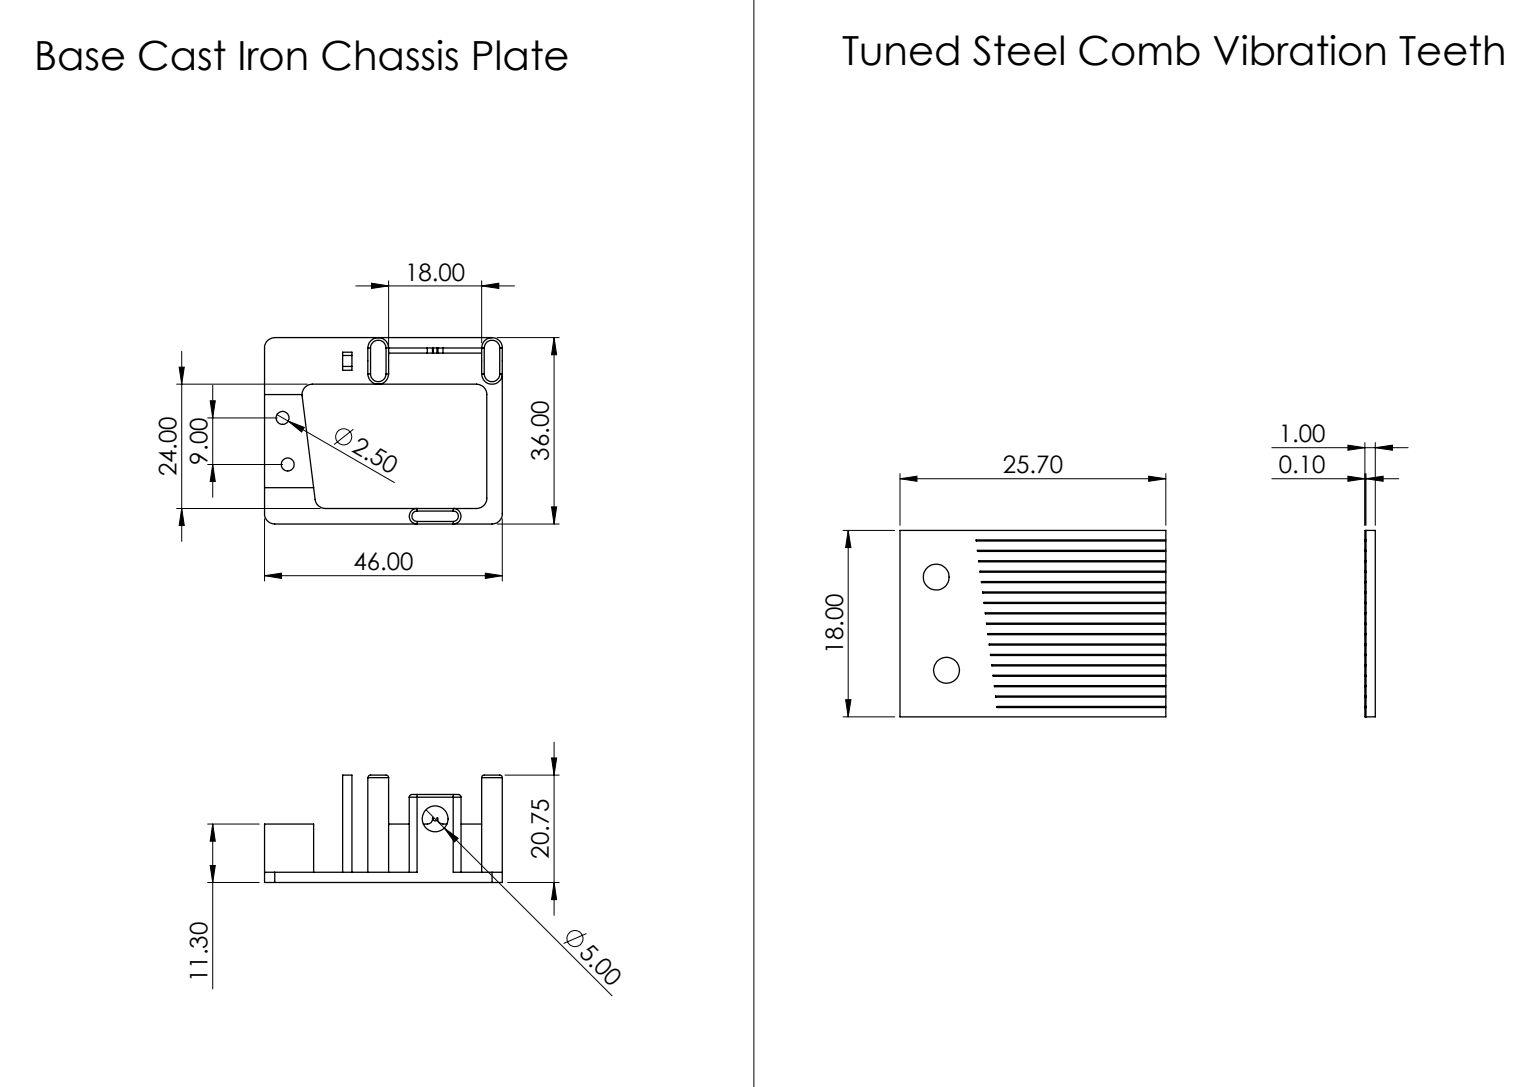
ISO-10303-21;
HEADER;
FILE_DESCRIPTION (('STEP AP214'),
    '1' );
FILE_NAME ('Tuned Steel Comb Vibration Teeth.step',
    '2026-10-09T09:51:18',
    ( '' ),
    ( '' ),
    'SwSTEP 2.0',
    'SolidWorks 2026',
    '' );
FILE_SCHEMA (( 'AUTOMOTIVE_DESIGN' ));
ENDSEC;

DATA;
#16=PLANE ( 'NONE',  #21145 ) ;
#64=LINE ( 'NONE', #7461, #9828 ) ;
#76=MANIFOLD_SOLID_BREP ( 'Stock-MAS-175-1', #12603 ) ;
#123=AXIS2_PLACEMENT_3D ( 'NONE', #20425, #35422, #737 ) ;
#135=ORIENTED_EDGE ( 'NONE', *, *, #41849, .T. ) ;
#167=CARTESIAN_POINT ( 'NONE',  ( -24.72409385541305582, -14.80920654474425291, 71.08235294117645253 ) ) ;
#180=DIRECTION ( 'NONE',  ( -2.866981220435666553E-17, 1.000000000000000000, 1.190614954331866791E-16 ) ) ;
#185=ORIENTED_EDGE ( 'NONE', *, *, #14224, .F. ) ;
#205=VERTEX_POINT ( 'NONE', #7298 ) ;
#229=ORIENTED_EDGE ( 'NONE', *, *, #12454, .F. ) ;
#252=ORIENTED_EDGE ( 'NONE', *, *, #29570, .F. ) ;
#261=PLANE ( 'NONE',  #46906 ) ;
#307=FACE_OUTER_BOUND ( 'NONE', #29969, .T. ) ;
#310=FACE_OUTER_BOUND ( 'NONE', #34779, .T. ) ;
#312=CARTESIAN_POINT ( 'NONE',  ( -50.42609385541305755, -14.80920654474418008, 64.94117647058821774 ) ) ;
#316=ORIENTED_EDGE ( 'NONE', *, *, #24449, .T. ) ;
#347=EDGE_CURVE ( 'NONE', #38066, #30065, #19519, .T. ) ;
#430=DIRECTION ( 'NONE',  ( 2.866981220435666553E-17, -1.000000000000000000, -1.190614954331866791E-16 ) ) ;
#432=EDGE_CURVE ( 'NONE', #1919, #29759, #26919, .T. ) ;
#454=VERTEX_POINT ( 'NONE', #31574 ) ;
#509=PLANE ( 'NONE',  #15734 ) ;
#529=CARTESIAN_POINT ( 'NONE',  ( -24.72409385541305582, -14.80920654474428488, 74.99999999999998579 ) ) ;
#555=VECTOR ( 'NONE', #30468, 1000.000000000000000 ) ;
#570=EDGE_LOOP ( 'NONE', ( #41024, #28488, #8043, #46149 ) ) ;
#577=DIRECTION ( 'NONE',  ( 3.413470714839332458E-33, -1.190614954331866791E-16, 1.000000000000000000 ) ) ;
#581=DIRECTION ( 'NONE',  ( -1.000000000000000000, -2.866981220435666553E-17, -0.000000000000000000 ) ) ;
#589=FACE_OUTER_BOUND ( 'NONE', #44283, .T. ) ;
#629=DIRECTION ( 'NONE',  ( -2.866981220435666553E-17, 1.000000000000000000, 1.190614954331866791E-16 ) ) ;
#653=LINE ( 'NONE', #19120, #11762 ) ;
#659=LINE ( 'NONE', #18884, #6970 ) ;
#660=CARTESIAN_POINT ( 'NONE',  ( -43.16186218120491702, -14.90920654474411577, 57.09785339366514734 ) ) ;
#663=EDGE_CURVE ( 'NONE', #29482, #47620, #41570, .T. ) ;
#665=ORIENTED_EDGE ( 'NONE', *, *, #5113, .F. ) ;
#721=CARTESIAN_POINT ( 'NONE',  ( -24.72409385541305582, -14.80920654474417830, 64.04117647058822627 ) ) ;
#732=CARTESIAN_POINT ( 'NONE',  ( -50.42609385541305755, -14.90920654474416907, 63.03529411764704804 ) ) ;
#737=DIRECTION ( 'NONE',  ( -2.866981220435666553E-17, 1.000000000000000000, 1.190614954331866791E-16 ) ) ;
#738=CARTESIAN_POINT ( 'NONE',  ( -50.42609385541305755, -14.90920654474420104, 66.95294117647057419 ) ) ;
#757=DIRECTION ( 'NONE',  ( -1.000000000000000000, -2.866981220435666553E-17, 0.000000000000000000 ) ) ;
#764=CARTESIAN_POINT ( 'NONE',  ( -24.72409385541305582, -14.80920654474425291, 71.98235294117645822 ) ) ;
#790=PLANE ( 'NONE',  #17368 ) ;
#815=VECTOR ( 'NONE', #1897, 1000.000000000000000 ) ;
#864=DIRECTION ( 'NONE',  ( -2.866981220435666553E-17, 1.000000000000000000, 1.190614954331866791E-16 ) ) ;
#896=CARTESIAN_POINT ( 'NONE',  ( -24.72409385541305582, -14.80920654474425291, 71.08235294117645253 ) ) ;
#901=EDGE_LOOP ( 'NONE', ( #45786, #21346, #14320, #44685 ) ) ;
#950=CARTESIAN_POINT ( 'NONE',  ( -24.72409385541305582, -15.80920654474410725, 65.99999999999998579 ) ) ;
#954=EDGE_CURVE ( 'NONE', #6612, #48084, #29451, .T. ) ;
#958=AXIS2_PLACEMENT_3D ( 'NONE', #45857, #23205, #45623 ) ;
#970=DIRECTION ( 'NONE',  ( -2.866981220435666553E-17, 1.000000000000000000, 1.190614954331866791E-16 ) ) ;
#1025=DIRECTION ( 'NONE',  ( -0.1240347345892086200, 1.145860353393066553E-16, -0.9922778767136676281 ) ) ;
#1043=VECTOR ( 'NONE', #24003, 1000.000000000000000 ) ;
#1070=ORIENTED_EDGE ( 'NONE', *, *, #26487, .T. ) ;
#1101=AXIS2_PLACEMENT_3D ( 'NONE', #39404, #35686, #5686 ) ;
#1104=CARTESIAN_POINT ( 'NONE',  ( -50.42609385541305755, -14.90920654474421170, 67.05882352941175384 ) ) ;
#1107=EDGE_CURVE ( 'NONE', #11974, #16121, #19840, .T. ) ;
#1125=LINE ( 'NONE', #31171, #38141 ) ;
#1160=LINE ( 'NONE', #26797, #17877 ) ;
#1164=CARTESIAN_POINT ( 'NONE',  ( -24.72409385541305582, -14.80920654474424225, 70.97647058823527288 ) ) ;
#1212=EDGE_CURVE ( 'NONE', #47915, #46865, #47396, .T. ) ;
#1241=ORIENTED_EDGE ( 'NONE', *, *, #1212, .T. ) ;
#1245=CARTESIAN_POINT ( 'NONE',  ( -43.04835856129541583, -14.80920654474411613, 58.00588235294116402 ) ) ;
#1252=LINE ( 'NONE', #16256, #44627 ) ;
#1269=DIRECTION ( 'NONE',  ( -2.866981220435666553E-17, 1.000000000000000000, 1.190614954331866791E-16 ) ) ;
#1304=LINE ( 'NONE', #23249, #38376 ) ;
#1329=DIRECTION ( 'NONE',  ( -2.866981220435666553E-17, 1.000000000000000000, 1.190614954331866791E-16 ) ) ;
#1332=ORIENTED_EDGE ( 'NONE', *, *, #40037, .F. ) ;
#1372=VECTOR ( 'NONE', #42277, 1000.000000000000000 ) ;
#1374=VERTEX_POINT ( 'NONE', #19527 ) ;
#1381=DIRECTION ( 'NONE',  ( -3.413470714839332458E-33, 1.190614954331866791E-16, -1.000000000000000000 ) ) ;
#1410=VERTEX_POINT ( 'NONE', #34789 ) ;
#1420=VERTEX_POINT ( 'NONE', #4273 ) ;
#1430=PLANE ( 'NONE',  #34332 ) ;
#1455=LINE ( 'NONE', #16465, #14102 ) ;
#1487=EDGE_CURVE ( 'NONE', #15891, #24038, #38965, .T. ) ;
#1515=AXIS2_PLACEMENT_3D ( 'NONE', #48179, #29470, #40541 ) ;
#1548=VECTOR ( 'NONE', #1329, 1000.000000000000000 ) ;
#1561=EDGE_CURVE ( 'NONE', #1863, #1410, #13329, .T. ) ;
#1579=DIRECTION ( 'NONE',  ( -3.652049423109068320E-16, 1.190614954331866791E-16, -1.000000000000000000 ) ) ;
#1620=EDGE_CURVE ( 'NONE', #2135, #40793, #37425, .T. ) ;
#1626=CARTESIAN_POINT ( 'NONE',  ( -42.18144679658952612, -14.80920654474417830, 64.94117647058821774 ) ) ;
#1641=EDGE_CURVE ( 'NONE', #46610, #24230, #44142, .T. ) ;
#1647=VECTOR ( 'NONE', #12531, 1000.000000000000000 ) ;
#1662=VERTEX_POINT ( 'NONE', #29574 ) ;
#1679=VECTOR ( 'NONE', #28191, 1000.000000000000000 ) ;
#1680=ORIENTED_EDGE ( 'NONE', *, *, #28119, .F. ) ;
#1684=DIRECTION ( 'NONE',  ( -2.866981220435666553E-17, 1.000000000000000000, 1.190614954331866791E-16 ) ) ;
#1727=DIRECTION ( 'NONE',  ( 1.000000000000000000, 2.866981220435666553E-17, 0.000000000000000000 ) ) ;
#1815=PLANE ( 'NONE',  #25993 ) ;
#1863=VERTEX_POINT ( 'NONE', #35927 ) ;
#1889=EDGE_CURVE ( 'NONE', #47208, #6712, #40360, .T. ) ;
#1892=DIRECTION ( 'NONE',  ( 1.000000000000000000, 2.866981220435666553E-17, 0.000000000000000000 ) ) ;
#1897=DIRECTION ( 'NONE',  ( 3.413470714839332458E-33, -1.190614954331866791E-16, 1.000000000000000000 ) ) ;
#1910=ORIENTED_EDGE ( 'NONE', *, *, #27558, .F. ) ;
#1915=EDGE_CURVE ( 'NONE', #40821, #18743, #40128, .T. ) ;
#1916=EDGE_CURVE ( 'NONE', #45934, #39678, #17693, .T. ) ;
#1917=VECTOR ( 'NONE', #12087, 1000.000000000000000 ) ;
#1919=VERTEX_POINT ( 'NONE', #2920 ) ;
#1944=VECTOR ( 'NONE', #14922, 1000.000000000000000 ) ;
#1945=CARTESIAN_POINT ( 'NONE',  ( -43.28566308618228931, -14.90920654474410512, 56.10744615384614065 ) ) ;
#1970=EDGE_CURVE ( 'NONE', #1420, #21415, #44084, .T. ) ;
#1984=VECTOR ( 'NONE', #8791, 1000.000000000000000 ) ;
#2003=FACE_OUTER_BOUND ( 'NONE', #7911, .T. ) ;
#2007=ORIENTED_EDGE ( 'NONE', *, *, #19882, .T. ) ;
#2017=FACE_OUTER_BOUND ( 'NONE', #3231, .T. ) ;
#2032=EDGE_CURVE ( 'NONE', #25220, #35234, #33938, .T. ) ;
#2077=ADVANCED_FACE ( 'NONE', ( #8584 ), #41836, .F. ) ;
#2110=VERTEX_POINT ( 'NONE', #38350 ) ;
#2120=VECTOR ( 'NONE', #27838, 1000.000000000000000 ) ;
#2135=VERTEX_POINT ( 'NONE', #38612 ) ;
#2137=FACE_OUTER_BOUND ( 'NONE', #36078, .T. ) ;
#2150=VECTOR ( 'NONE', #9834, 1000.000000000000000 ) ;
#2169=CARTESIAN_POINT ( 'NONE',  ( -41.91674091423659121, -14.90920654474421170, 67.05882352941175384 ) ) ;
#2179=VECTOR ( 'NONE', #10449, 1000.000000000000000 ) ;
#2253=CIRCLE ( 'NONE', #29790, 1.250000000000001110 ) ;
#2263=CARTESIAN_POINT ( 'NONE',  ( -50.42409385541305511, -15.80920654474410725, 74.99999999999998579 ) ) ;
#2265=LINE ( 'NONE', #23962, #17172 ) ;
#2281=CARTESIAN_POINT ( 'NONE',  ( -50.42609385541305755, -14.80920654474415699, 62.92941176470587550 ) ) ;
#2286=CARTESIAN_POINT ( 'NONE',  ( -50.42609385541305755, -14.80920654474415699, 62.02941176470587692 ) ) ;
#2333=CARTESIAN_POINT ( 'NONE',  ( -24.72409385541305582, -14.90920654474417972, 64.04117647058822627 ) ) ;
#2361=VECTOR ( 'NONE', #13653, 1000.000000000000000 ) ;
#2362=ORIENTED_EDGE ( 'NONE', *, *, #2957, .F. ) ;
#2368=DIRECTION ( 'NONE',  ( 2.866981220435666553E-17, -1.000000000000000000, -1.190614954331866791E-16 ) ) ;
#2379=ORIENTED_EDGE ( 'NONE', *, *, #11206, .F. ) ;
#2398=ORIENTED_EDGE ( 'NONE', *, *, #23944, .T. ) ;
#2416=ORIENTED_EDGE ( 'NONE', *, *, #36323, .T. ) ;
#2418=STYLED_ITEM ( 'NONE', ( #3339 ), #76 ) ;
#2429=AXIS2_PLACEMENT_3D ( 'NONE', #45470, #44997, #11245 ) ;
#2435=LINE ( 'NONE', #40111, #21168 ) ;
#2451=LINE ( 'NONE', #13984, #22078 ) ;
#2455=ORIENTED_EDGE ( 'NONE', *, *, #40556, .T. ) ;
#2466=CARTESIAN_POINT ( 'NONE',  ( -50.42609385541305755, -14.80920654474412679, 59.01176470588234224 ) ) ;
#2476=AXIS2_PLACEMENT_3D ( 'NONE', #39433, #5710, #32041 ) ;
#2478=DIRECTION ( 'NONE',  ( 3.413470714839332458E-33, -1.190614954331866791E-16, 1.000000000000000000 ) ) ;
#2485=PLANE ( 'NONE',  #37833 ) ;
#2502=ADVANCED_FACE ( 'NONE', ( #47100 ), #32330, .T. ) ;
#2509=VECTOR ( 'NONE', #12897, 1000.000000000000000 ) ;
#2553=CARTESIAN_POINT ( 'NONE',  ( -50.42609385541305755, -14.80920654474427600, 73.99411764705880046 ) ) ;
#2593=ORIENTED_EDGE ( 'NONE', *, *, #18017, .F. ) ;
#2594=VECTOR ( 'NONE', #6001, 1000.000000000000000 ) ;
#2611=LINE ( 'NONE', #29437, #43798 ) ;
#2661=EDGE_CURVE ( 'NONE', #8589, #29913, #45118, .T. ) ;
#2705=EDGE_CURVE ( 'NONE', #6966, #37287, #34488, .T. ) ;
#2721=ORIENTED_EDGE ( 'NONE', *, *, #3390, .T. ) ;
#2727=EDGE_LOOP ( 'NONE', ( #16534, #10363, #44094, #48223 ) ) ;
#2731=ORIENTED_EDGE ( 'NONE', *, *, #14015, .F. ) ;
#2744=DIRECTION ( 'NONE',  ( -2.866981220435666553E-17, 1.000000000000000000, 1.190614954331866791E-16 ) ) ;
#2749=ORIENTED_EDGE ( 'NONE', *, *, #45902, .F. ) ;
#2769=DIRECTION ( 'NONE',  ( 3.413470714839332458E-33, -1.190614954331866791E-16, 1.000000000000000000 ) ) ;
#2801=DIRECTION ( 'NONE',  ( 1.000000000000000000, 0.000000000000000000, 0.000000000000000000 ) ) ;
#2808=FACE_OUTER_BOUND ( 'NONE', #43285, .T. ) ;
#2823=LINE ( 'NONE', #29420, #2361 ) ;
#2862=DIRECTION ( 'NONE',  ( 3.413470714839332458E-33, -1.190614954331866791E-16, 1.000000000000000000 ) ) ;
#2880=CARTESIAN_POINT ( 'NONE',  ( -50.42409385541305511, -15.80920654474410725, 56.99999999999998579 ) ) ;
#2904=ORIENTED_EDGE ( 'NONE', *, *, #28510, .F. ) ;
#2916=EDGE_LOOP ( 'NONE', ( #37319, #22808, #28235, #38298 ) ) ;
#2920=CARTESIAN_POINT ( 'NONE',  ( -24.72409385541305582, -14.80920654474415699, 62.02941176470587692 ) ) ;
#2927=EDGE_CURVE ( 'NONE', #30495, #47915, #33684, .T. ) ;
#2951=VECTOR ( 'NONE', #21534, 1000.000000000000000 ) ;
#2957=EDGE_CURVE ( 'NONE', #15234, #24799, #48719, .T. ) ;
#2973=AXIS2_PLACEMENT_3D ( 'NONE', #33729, #30074, #19219 ) ;
#2996=FACE_OUTER_BOUND ( 'NONE', #30465, .T. ) ;
#3005=DIRECTION ( 'NONE',  ( 3.413470714839332458E-33, -1.190614954331866791E-16, 1.000000000000000000 ) ) ;
#3025=CIRCLE ( 'NONE', #8564, 1.250000000000001110 ) ;
#3027=EDGE_LOOP ( 'NONE', ( #18259, #31844, #3708, #42426 ) ) ;
#3098=DIRECTION ( 'NONE',  ( -2.866981220435666553E-17, 1.000000000000000000, 1.190614954331866791E-16 ) ) ;
#3104=EDGE_CURVE ( 'NONE', #3303, #10012, #18937, .T. ) ;
#3144=ORIENTED_EDGE ( 'NONE', *, *, #17911, .T. ) ;
#3161=VECTOR ( 'NONE', #37100, 1000.000000000000000 ) ;
#3164=LINE ( 'NONE', #17455, #12414 ) ;
#3169=EDGE_CURVE ( 'NONE', #22665, #37829, #32209, .T. ) ;
#3208=CARTESIAN_POINT ( 'NONE',  ( -50.42609385541305755, -14.80920654474425291, 71.98235294117645822 ) ) ;
#3214=DIRECTION ( 'NONE',  ( 1.000000000000000000, 2.866981220435666553E-17, 0.000000000000000000 ) ) ;
#3231=EDGE_LOOP ( 'NONE', ( #25717, #29584, #23934, #15651 ) ) ;
#3238=CARTESIAN_POINT ( 'NONE',  ( -41.66527032600129843, -14.90920654474423124, 69.07058823529411029 ) ) ;
#3255=ADVANCED_FACE ( 'NONE', ( #42808 ), #9082, .T. ) ;
#3286=ORIENTED_EDGE ( 'NONE', *, *, #36696, .T. ) ;
#3296=DIRECTION ( 'NONE',  ( -1.000000000000000000, -2.866981220435666553E-17, -0.000000000000000000 ) ) ;
#3303=VERTEX_POINT ( 'NONE', #36592 ) ;
#3312=ORIENTED_EDGE ( 'NONE', *, *, #25292, .T. ) ;
#3324=CARTESIAN_POINT ( 'NONE',  ( -42.93585856129541156, -14.90920654474411577, 58.90588235294116970 ) ) ;
#3332=EDGE_CURVE ( 'NONE', #17746, #11974, #25307, .T. ) ;
#3334=LINE ( 'NONE', #4321, #34343 ) ;
#3339=PRESENTATION_STYLE_ASSIGNMENT (( #5661 ) ) ;
#3390=EDGE_CURVE ( 'NONE', #39596, #18661, #11491, .T. ) ;
#3398=ADVANCED_FACE ( 'NONE', ( #4126 ), #19125, .F. ) ;
#3414=LINE ( 'NONE', #33192, #43322 ) ;
#3420=CARTESIAN_POINT ( 'NONE',  ( -24.72409385541305582, -14.90920654474427565, 73.99411764705880046 ) ) ;
#3443=DIRECTION ( 'NONE',  ( 3.413470714839332458E-33, -1.190614954331866791E-16, 1.000000000000000000 ) ) ;
#3447=VECTOR ( 'NONE', #36524, 1000.000000000000000 ) ;
#3476=LINE ( 'NONE', #45114, #3564 ) ;
#3528=CARTESIAN_POINT ( 'NONE',  ( -24.72409385541305582, -14.90920654474428630, 74.99999999999998579 ) ) ;
#3544=EDGE_CURVE ( 'NONE', #29528, #40648, #7040, .T. ) ;
#3564=VECTOR ( 'NONE', #14522, 1000.000000000000114 ) ;
#3587=LINE ( 'NONE', #167, #7934 ) ;
#3638=EDGE_CURVE ( 'NONE', #36414, #48232, #2611, .T. ) ;
#3663=CIRCLE ( 'NONE', #11509, 1.250000000000001110 ) ;
#3692=EDGE_CURVE ( 'NONE', #10012, #40467, #3334, .T. ) ;
#3696=DIRECTION ( 'NONE',  ( 1.000000000000000000, 2.866981220435666553E-17, 0.000000000000000000 ) ) ;
#3708=ORIENTED_EDGE ( 'NONE', *, *, #26564, .T. ) ;
#3711=ORIENTED_EDGE ( 'NONE', *, *, #28339, .F. ) ;
#3716=PLANE ( 'NONE',  #43067 ) ;
#3727=EDGE_CURVE ( 'NONE', #24420, #15891, #29934, .T. ) ;
#3733=ORIENTED_EDGE ( 'NONE', *, *, #25222, .T. ) ;
#3774=AXIS2_PLACEMENT_3D ( 'NONE', #35735, #38041, #8940 ) ;
#3790=DIRECTION ( 'NONE',  ( -3.413470714839332458E-33, 1.190614954331866791E-16, -1.000000000000000000 ) ) ;
#3806=ORIENTED_EDGE ( 'NONE', *, *, #9765, .T. ) ;
#3810=VECTOR ( 'NONE', #13222, 1000.000000000000000 ) ;
#3814=VECTOR ( 'NONE', #9796, 1000.000000000000000 ) ;
#3886=EDGE_CURVE ( 'NONE', #42514, #2110, #20305, .T. ) ;
#3919=VECTOR ( 'NONE', #19701, 1000.000000000000000 ) ;
#3945=CARTESIAN_POINT ( 'NONE',  ( -41.92997620835424044, -14.80920654474420139, 66.95294117647057419 ) ) ;
#3952=ORIENTED_EDGE ( 'NONE', *, *, #45569, .T. ) ;
#3961=EDGE_CURVE ( 'NONE', #3303, #19706, #44194, .T. ) ;
#3977=ADVANCED_FACE ( 'NONE', ( #17320 ), #17562, .T. ) ;
#3984=EDGE_LOOP ( 'NONE', ( #16935, #43466, #37026, #20839 ) ) ;
#3996=AXIS2_PLACEMENT_3D ( 'NONE', #37215, #19927, #22466 ) ;
#4004=DIRECTION ( 'NONE',  ( 2.866981220435666553E-17, -1.000000000000000000, -1.190614954331866791E-16 ) ) ;
#4005=LINE ( 'NONE', #30357, #14266 ) ;
#4029=EDGE_LOOP ( 'NONE', ( #6997, #34854, #3733, #46267 ) ) ;
#4030=DIRECTION ( 'NONE',  ( 1.000000000000000000, 2.866981220435666553E-17, 0.000000000000000000 ) ) ;
#4035=LINE ( 'NONE', #26680, #15536 ) ;
#4052=VECTOR ( 'NONE', #4155, 1000.000000000000000 ) ;
#4065=DIRECTION ( 'NONE',  ( 2.866981220435666553E-17, -1.000000000000000000, -1.190614954331866791E-16 ) ) ;
#4073=VECTOR ( 'NONE', #48266, 1000.000000000000000 ) ;
#4074=ORIENTED_EDGE ( 'NONE', *, *, #30635, .T. ) ;
#4113=CARTESIAN_POINT ( 'NONE',  ( -42.30718209070717961, -14.80920654474416764, 63.93529411764704662 ) ) ;
#4115=FACE_OUTER_BOUND ( 'NONE', #30233, .T. ) ;
#4126=FACE_OUTER_BOUND ( 'NONE', #42816, .T. ) ;
#4136=EDGE_CURVE ( 'NONE', #46865, #24126, #45385, .T. ) ;
#4140=ORIENTED_EDGE ( 'NONE', *, *, #45296, .F. ) ;
#4155=DIRECTION ( 'NONE',  ( 1.000000000000000000, 2.866981220435666553E-17, 0.000000000000000000 ) ) ;
#4188=LINE ( 'NONE', #19685, #17876 ) ;
#4191=LINE ( 'NONE', #34934, #1647 ) ;
#4209=CARTESIAN_POINT ( 'NONE',  ( -45.92409385541305511, -14.80920654474410725, 70.50000000000000000 ) ) ;
#4219=DIRECTION ( 'NONE',  ( 3.413470714839332458E-33, -1.190614954331866791E-16, 1.000000000000000000 ) ) ;
#4231=ORIENTED_EDGE ( 'NONE', *, *, #1889, .T. ) ;
#4260=ORIENTED_EDGE ( 'NONE', *, *, #44885, .T. ) ;
#4273=CARTESIAN_POINT ( 'NONE',  ( -41.16232914953070576, -14.80920654474410725, 73.09411764705880898 ) ) ;
#4319=FACE_OUTER_BOUND ( 'NONE', #43939, .T. ) ;
#4321=CARTESIAN_POINT ( 'NONE',  ( -24.72409385541305582, -14.90920654474421170, 67.05882352941175384 ) ) ;
#4322=ORIENTED_EDGE ( 'NONE', *, *, #48349, .F. ) ;
#4330=CARTESIAN_POINT ( 'NONE',  ( -24.72409385541305582, -14.90920654474424190, 70.07647058823528141 ) ) ;
#4344=ORIENTED_EDGE ( 'NONE', *, *, #32984, .T. ) ;
#4352=ORIENTED_EDGE ( 'NONE', *, *, #1107, .T. ) ;
#4427=EDGE_CURVE ( 'NONE', #21415, #46626, #33226, .T. ) ;
#4433=CARTESIAN_POINT ( 'NONE',  ( -50.42609385541305755, -14.80920654474423159, 69.07058823529411029 ) ) ;
#4442=DIRECTION ( 'NONE',  ( 2.866981220435666553E-17, -1.000000000000000000, -1.190614954331866791E-16 ) ) ;
#4443=PLANE ( 'NONE',  #30508 ) ;
#4458=DIRECTION ( 'NONE',  ( 2.866981220435666553E-17, -1.000000000000000000, -1.190614954331866791E-16 ) ) ;
#4555=ADVANCED_FACE ( 'NONE', ( #30555 ), #12788, .T. ) ;
#4565=ORIENTED_EDGE ( 'NONE', *, *, #34020, .T. ) ;
#4590=VERTEX_POINT ( 'NONE', #30798 ) ;
#4595=DIRECTION ( 'NONE',  ( -0.1240347345892086200, 1.145860353393066553E-16, -0.9922778767136676281 ) ) ;
#4611=VECTOR ( 'NONE', #6391, 1000.000000000000000 ) ;
#4659=AXIS2_PLACEMENT_3D ( 'NONE', #24925, #6214, #21235 ) ;
#4707=VECTOR ( 'NONE', #28793, 1000.000000000000000 ) ;
#4734=ORIENTED_EDGE ( 'NONE', *, *, #3692, .F. ) ;
#4807=ORIENTED_EDGE ( 'NONE', *, *, #22365, .T. ) ;
#4839=VERTEX_POINT ( 'NONE', #46899 ) ;
#4875=ORIENTED_EDGE ( 'NONE', *, *, #18257, .T. ) ;
#4891=ORIENTED_EDGE ( 'NONE', *, *, #1487, .F. ) ;
#4895=DIRECTION ( 'NONE',  ( 2.866981220435666553E-17, -1.000000000000000000, -1.190614954331866791E-16 ) ) ;
#4907=CARTESIAN_POINT ( 'NONE',  ( -50.42409385541305511, -15.80920654474410725, 56.99999999999998579 ) ) ;
#4937=DIRECTION ( 'NONE',  ( -2.866981220435666553E-17, 1.000000000000000000, 1.190614954331866791E-16 ) ) ;
#4975=CARTESIAN_POINT ( 'NONE',  ( -24.72409385541305582, -14.90920654474421170, 67.05882352941175384 ) ) ;
#4985=EDGE_CURVE ( 'NONE', #29698, #14925, #25223, .T. ) ;
#4990=VECTOR ( 'NONE', #20067, 1000.000000000000000 ) ;
#5059=EDGE_CURVE ( 'NONE', #37287, #30155, #23233, .T. ) ;
#5082=ORIENTED_EDGE ( 'NONE', *, *, #14082, .T. ) ;
#5084=ORIENTED_EDGE ( 'NONE', *, *, #27009, .F. ) ;
#5090=ORIENTED_EDGE ( 'NONE', *, *, #35204, .F. ) ;
#5094=AXIS2_PLACEMENT_3D ( 'NONE', #2281, #13586, #17288 ) ;
#5113=EDGE_CURVE ( 'NONE', #10119, #6712, #4035, .T. ) ;
#5128=CARTESIAN_POINT ( 'NONE',  ( -42.18144679658953322, -14.80920654474417830, 64.94117647058821774 ) ) ;
#5144=CARTESIAN_POINT ( 'NONE',  ( -40.92409385541305511, -14.80920654474410725, 74.99999999999998579 ) ) ;
#5178=ORIENTED_EDGE ( 'NONE', *, *, #27558, .T. ) ;
#5199=CARTESIAN_POINT ( 'NONE',  ( -24.72409385541305582, -14.80920654474426357, 72.98823529411762934 ) ) ;
#5210=ADVANCED_FACE ( 'NONE', ( #5490 ), #16293, .T. ) ;
#5222=VECTOR ( 'NONE', #23113, 1000.000000000000000 ) ;
#5224=ORIENTED_EDGE ( 'NONE', *, *, #5938, .T. ) ;
#5235=DIRECTION ( 'NONE',  ( 1.000000000000000000, 0.000000000000000000, 0.000000000000000000 ) ) ;
#5242=ORIENTED_EDGE ( 'NONE', *, *, #17838, .F. ) ;
#5267=ADVANCED_FACE ( 'NONE', ( #36684 ), #28612, .T. ) ;
#5285=LINE ( 'NONE', #17066, #13109 ) ;
#5333=EDGE_CURVE ( 'NONE', #46610, #32982, #44139, .T. ) ;
#5362=ORIENTED_EDGE ( 'NONE', *, *, #44509, .T. ) ;
#5370=ORIENTED_EDGE ( 'NONE', *, *, #36392, .T. ) ;
#5401=CIRCLE ( 'NONE', #10106, 1.250000000000001110 ) ;
#5402=ORIENTED_EDGE ( 'NONE', *, *, #13893, .F. ) ;
#5412=( LENGTH_UNIT ( ) NAMED_UNIT ( * ) SI_UNIT ( .MILLI., .METRE. ) );
#5448=VECTOR ( 'NONE', #24917, 1000.000000000000000 ) ;
#5490=FACE_OUTER_BOUND ( 'NONE', #47453, .T. ) ;
#5517=VECTOR ( 'NONE', #15046, 1000.000000000000000 ) ;
#5522=DIRECTION ( 'NONE',  ( -2.866981220435666553E-17, 1.000000000000000000, 1.190614954331866791E-16 ) ) ;
#5572=EDGE_LOOP ( 'NONE', ( #5896, #24563, #3952, #26022 ) ) ;
#5607=VERTEX_POINT ( 'NONE', #12260 ) ;
#5630=CARTESIAN_POINT ( 'NONE',  ( -42.43291738482482600, -14.80920654474415699, 62.92941176470587550 ) ) ;
#5637=CARTESIAN_POINT ( 'NONE',  ( -50.42609385541305755, -14.80920654474424225, 70.07647058823528141 ) ) ;
#5661=SURFACE_STYLE_USAGE ( .BOTH. , #37057 ) ;
#5667=ORIENTED_EDGE ( 'NONE', *, *, #8161, .F. ) ;
#5677=ORIENTED_EDGE ( 'NONE', *, *, #41950, .F. ) ;
#5686=DIRECTION ( 'NONE',  ( 1.000000000000000000, 0.000000000000000000, 0.000000000000000000 ) ) ;
#5688=ORIENTED_EDGE ( 'NONE', *, *, #38380, .F. ) ;
#5710=DIRECTION ( 'NONE',  ( -3.413470714839332458E-33, 1.190614954331866791E-16, -1.000000000000000000 ) ) ;
#5712=EDGE_CURVE ( 'NONE', #38928, #19353, #10996, .T. ) ;
#5720=LINE ( 'NONE', #20728, #16300 ) ;
#5734=CARTESIAN_POINT ( 'NONE',  ( -50.42609385541305755, -14.80920654474414810, 61.02352941176469869 ) ) ;
#5760=EDGE_LOOP ( 'NONE', ( #19411, #44640, #8100, #24991 ) ) ;
#5790=EDGE_CURVE ( 'NONE', #12016, #40648, #25520, .T. ) ;
#5795=LINE ( 'NONE', #20804, #21278 ) ;
#5804=LINE ( 'NONE', #9741, #18191 ) ;
#5815=FACE_BOUND ( 'NONE', #47142, .T. ) ;
#5841=ORIENTED_EDGE ( 'NONE', *, *, #2705, .F. ) ;
#5878=EDGE_CURVE ( 'NONE', #29913, #1863, #8056, .T. ) ;
#5896=ORIENTED_EDGE ( 'NONE', *, *, #17120, .F. ) ;
#5897=LINE ( 'NONE', #17920, #20475 ) ;
#5910=CARTESIAN_POINT ( 'NONE',  ( -41.66527032600129132, -14.80920654474410725, 69.07058823529411029 ) ) ;
#5926=ORIENTED_EDGE ( 'NONE', *, *, #10220, .F. ) ;
#5938=EDGE_CURVE ( 'NONE', #41531, #29759, #39461, .T. ) ;
#5939=LINE ( 'NONE', #47314, #47305 ) ;
#5949=ORIENTED_EDGE ( 'NONE', *, *, #22285, .T. ) ;
#5954=ORIENTED_EDGE ( 'NONE', *, *, #40077, .F. ) ;
#5975=PLANE ( 'NONE',  #5094 ) ;
#5993=ORIENTED_EDGE ( 'NONE', *, *, #28984, .T. ) ;
#6001=DIRECTION ( 'NONE',  ( 3.413470714839332458E-33, -1.190614954331866791E-16, 1.000000000000000000 ) ) ;
#6016=DIRECTION ( 'NONE',  ( -2.866981220435666553E-17, 1.000000000000000000, 1.190614954331866791E-16 ) ) ;
#6018=EDGE_LOOP ( 'NONE', ( #2379, #40890, #14152, #35053 ) ) ;
#6027=DIRECTION ( 'NONE',  ( -2.866981220435666553E-17, 1.000000000000000000, 1.190614954331866791E-16 ) ) ;
#6037=ORIENTED_EDGE ( 'NONE', *, *, #47973, .F. ) ;
#6054=ADVANCED_FACE ( 'NONE', ( #40188 ), #6460, .T. ) ;
#6058=ORIENTED_EDGE ( 'NONE', *, *, #1641, .T. ) ;
#6147=DIRECTION ( 'NONE',  ( -2.866981220435666553E-17, 1.000000000000000000, 1.190614954331866791E-16 ) ) ;
#6175=CARTESIAN_POINT ( 'NONE',  ( -50.42609385541305755, -14.80920654474421205, 67.95882352941174531 ) ) ;
#6181=ORIENTED_EDGE ( 'NONE', *, *, #14611, .T. ) ;
#6200=EDGE_CURVE ( 'NONE', #40467, #23280, #26374, .T. ) ;
#6214=DIRECTION ( 'NONE',  ( -1.000000000000000000, -2.866981220435666553E-17, 0.000000000000000000 ) ) ;
#6221=CARTESIAN_POINT ( 'NONE',  ( -50.42609385541305755, -14.90920654474410512, 56.99999999999998579 ) ) ;
#6226=EDGE_LOOP ( 'NONE', ( #15030, #18307, #15418, #35070 ) ) ;
#6308=ADVANCED_FACE ( 'NONE', ( #30818 ), #12089, .F. ) ;
#6309=ORIENTED_EDGE ( 'NONE', *, *, #27193, .F. ) ;
#6363=VECTOR ( 'NONE', #13235, 1000.000000000000000 ) ;
#6391=DIRECTION ( 'NONE',  ( -3.413470714839332458E-33, 1.190614954331866791E-16, -1.000000000000000000 ) ) ;
#6460=PLANE ( 'NONE',  #13970 ) ;
#6464=ORIENTED_EDGE ( 'NONE', *, *, #36837, .F. ) ;
#6481=LINE ( 'NONE', #10420, #26660 ) ;
#6593=DIRECTION ( 'NONE',  ( 2.866981220435666553E-17, -1.000000000000000000, -1.190614954331866791E-16 ) ) ;
#6600=LINE ( 'NONE', #11021, #45659 ) ;
#6612=VERTEX_POINT ( 'NONE', #22065 ) ;
#6634=DIRECTION ( 'NONE',  ( -0.1240347345892086062, 1.145860353393066553E-16, -0.9922778767136676281 ) ) ;
#6655=VECTOR ( 'NONE', #25659, 1000.000000000000114 ) ;
#6657=CARTESIAN_POINT ( 'NONE',  ( -45.92409385541305511, -15.80920654474410725, 70.50000000000000000 ) ) ;
#6661=DIRECTION ( 'NONE',  ( 1.000000000000000000, 2.866981220435666553E-17, 0.000000000000000000 ) ) ;
#6675=DIRECTION ( 'NONE',  ( 1.000000000000000000, 2.866981220435666553E-17, 0.000000000000000000 ) ) ;
#6681=DIRECTION ( 'NONE',  ( -3.413470714839332458E-33, 1.190614954331866791E-16, -1.000000000000000000 ) ) ;
#6712=VERTEX_POINT ( 'NONE', #46666 ) ;
#6759=EDGE_CURVE ( 'NONE', #34260, #14295, #15880, .T. ) ;
#6795=ORIENTED_EDGE ( 'NONE', *, *, #14224, .T. ) ;
#6811=CARTESIAN_POINT ( 'NONE',  ( -42.54285765631804139, -14.90920654474416907, 62.04988959276017368 ) ) ;
#6829=DIRECTION ( 'NONE',  ( -1.000000000000000000, -2.866981220435666553E-17, -0.000000000000000000 ) ) ;
#6837=CARTESIAN_POINT ( 'NONE',  ( -50.42609385541305755, -14.90920654474428630, 74.09999999999998010 ) ) ;
#6863=CARTESIAN_POINT ( 'NONE',  ( -24.72409385541305582, -14.90920654474422058, 68.96470588235293064 ) ) ;
#6894=CARTESIAN_POINT ( 'NONE',  ( -48.17409385541305511, -14.80920654474410547, 61.49999999999999289 ) ) ;
#6896=ORIENTED_EDGE ( 'NONE', *, *, #34020, .F. ) ;
#6904=VECTOR ( 'NONE', #7689, 1000.000000000000114 ) ;
#6908=LINE ( 'NONE', #40881, #4073 ) ;
#6923=VECTOR ( 'NONE', #34977, 1000.000000000000114 ) ;
#6930=VECTOR ( 'NONE', #46243, 1000.000000000000000 ) ;
#6938=EDGE_CURVE ( 'NONE', #40783, #40793, #3025, .T. ) ;
#6945=VECTOR ( 'NONE', #45724, 1000.000000000000000 ) ;
#6956=CARTESIAN_POINT ( 'NONE',  ( -42.66665856129541368, -14.90920654474415841, 61.05948235294116699 ) ) ;
#6966=VERTEX_POINT ( 'NONE', #40965 ) ;
#6970=VECTOR ( 'NONE', #18618, 1000.000000000000000 ) ;
#6974=VERTEX_POINT ( 'NONE', #7494 ) ;
#6980=CARTESIAN_POINT ( 'NONE',  ( -41.55277032600130127, -14.80920654474423159, 69.97058823529410176 ) ) ;
#6992=CARTESIAN_POINT ( 'NONE',  ( -40.92409385541305511, -14.80920654474410725, 74.99999999999998579 ) ) ;
#6997=ORIENTED_EDGE ( 'NONE', *, *, #23807, .F. ) ;
#7006=VERTEX_POINT ( 'NONE', #3528 ) ;
#7010=AXIS2_PLACEMENT_3D ( 'NONE', #25113, #43838, #180 ) ;
#7013=ORIENTED_EDGE ( 'NONE', *, *, #39849, .T. ) ;
#7040=LINE ( 'NONE', #32175, #32760 ) ;
#7041=VECTOR ( 'NONE', #32205, 1000.000000000000000 ) ;
#7044=CARTESIAN_POINT ( 'NONE',  ( -44.67409385541304800, -15.81020654474410847, 70.50000000000000000 ) ) ;
#7058=ORIENTED_EDGE ( 'NONE', *, *, #23944, .F. ) ;
#7084=CARTESIAN_POINT ( 'NONE',  ( -50.42609385541305755, -14.90920654474426499, 72.08823529411763786 ) ) ;
#7106=EDGE_CURVE ( 'NONE', #42696, #22914, #23960, .T. ) ;
#7108=DIRECTION ( 'NONE',  ( 3.413470714839332458E-33, -1.190614954331866791E-16, 1.000000000000000000 ) ) ;
#7109=VECTOR ( 'NONE', #48034, 1000.000000000000000 ) ;
#7144=VERTEX_POINT ( 'NONE', #11908 ) ;
#7157=LINE ( 'NONE', #11823, #29190 ) ;
#7160=ORIENTED_EDGE ( 'NONE', *, *, #28024, .F. ) ;
#7188=CARTESIAN_POINT ( 'NONE',  ( -50.42609385541305755, -14.80920654474427600, 73.99411764705880046 ) ) ;
#7189=EDGE_LOOP ( 'NONE', ( #39531, #15160, #45984, #2593 ) ) ;
#7226=EDGE_CURVE ( 'NONE', #22495, #21028, #9903, .T. ) ;
#7290=LINE ( 'NONE', #25738, #43820 ) ;
#7298=CARTESIAN_POINT ( 'NONE',  ( -24.72409385541305582, -14.80920654474428488, 74.09999999999998010 ) ) ;
#7339=FACE_OUTER_BOUND ( 'NONE', #30283, .T. ) ;
#7399=VERTEX_POINT ( 'NONE', #5128 ) ;
#7417=DIRECTION ( 'NONE',  ( 2.866981220435666553E-17, -1.000000000000000000, -1.190614954331866791E-16 ) ) ;
#7432=CARTESIAN_POINT ( 'NONE',  ( -41.80424091423658695, -14.80920654474421205, 67.95882352941174531 ) ) ;
#7451=AXIS2_PLACEMENT_3D ( 'NONE', #45358, #38184, #11133 ) ;
#7461=CARTESIAN_POINT ( 'NONE',  ( -42.81012326717776517, -14.80920654474412679, 59.91176470588234793 ) ) ;
#7494=CARTESIAN_POINT ( 'NONE',  ( -42.04247620835423760, -14.90920654474420104, 66.05294117647058272 ) ) ;
#7498=CARTESIAN_POINT ( 'NONE',  ( -24.72409385541305582, -14.80920654474425291, 71.98235294117645822 ) ) ;
#7509=ORIENTED_EDGE ( 'NONE', *, *, #38603, .T. ) ;
#7553=DIRECTION ( 'NONE',  ( -2.866981220435666553E-17, 1.000000000000000000, 1.190614954331866791E-16 ) ) ;
#7568=DIRECTION ( 'NONE',  ( -2.866981220435666553E-17, 1.000000000000000000, 1.190614954331866791E-16 ) ) ;
#7591=AXIS2_PLACEMENT_3D ( 'NONE', #28532, #46758, #13002 ) ;
#7611=CARTESIAN_POINT ( 'NONE',  ( -42.16821150247189109, -14.90920654474419038, 65.04705882352939739 ) ) ;
#7629=ORIENTED_EDGE ( 'NONE', *, *, #47973, .T. ) ;
#7633=DIRECTION ( 'NONE',  ( 3.413470714839332458E-33, -1.190614954331866791E-16, 1.000000000000000000 ) ) ;
#7660=EDGE_CURVE ( 'NONE', #36955, #21913, #26501, .T. ) ;
#7670=VERTEX_POINT ( 'NONE', #4113 ) ;
#7671=LINE ( 'NONE', #23168, #23901 ) ;
#7689=DIRECTION ( 'NONE',  ( -0.1240347345892086062, 1.145860353393066553E-16, -0.9922778767136676281 ) ) ;
#7695=CARTESIAN_POINT ( 'NONE',  ( -40.92409385541305511, -14.80920654474410725, 74.99999999999998579 ) ) ;
#7707=LINE ( 'NONE', #312, #19748 ) ;
#7711=ORIENTED_EDGE ( 'NONE', *, *, #12560, .T. ) ;
#7730=CARTESIAN_POINT ( 'NONE',  ( -24.72409385541305582, -14.80920654474415699, 62.92941176470587550 ) ) ;
#7747=DIRECTION ( 'NONE',  ( 2.866981220435666553E-17, -1.000000000000000000, -1.190614954331866791E-16 ) ) ;
#7767=CARTESIAN_POINT ( 'NONE',  ( -42.16821150247188399, -14.80920654474410547, 65.04705882352939739 ) ) ;
#7768=VECTOR ( 'NONE', #44543, 1000.000000000000000 ) ;
#7783=EDGE_CURVE ( 'NONE', #22618, #8614, #30698, .T. ) ;
#7853=CARTESIAN_POINT ( 'NONE',  ( -50.42609385541305755, -14.80920654474411613, 58.00588235294116402 ) ) ;
#7872=EDGE_LOOP ( 'NONE', ( #38232, #31545, #46045, #25751 ) ) ;
#7878=VECTOR ( 'NONE', #23107, 1000.000000000000000 ) ;
#7893=LINE ( 'NONE', #3945, #42204 ) ;
#7911=EDGE_LOOP ( 'NONE', ( #33232, #9591, #12350, #47101 ) ) ;
#7925=LINE ( 'NONE', #764, #30606 ) ;
#7934=VECTOR ( 'NONE', #3098, 1000.000000000000000 ) ;
#7942=ADVANCED_FACE ( 'NONE', ( #25236 ), #21305, .F. ) ;
#7946=ADVANCED_FACE ( 'NONE', ( #2808 ), #32386, .T. ) ;
#7947=DIRECTION ( 'NONE',  ( 1.000000000000000000, 2.866981220435666553E-17, 0.000000000000000000 ) ) ;
#7953=CARTESIAN_POINT ( 'NONE',  ( -42.30718209070717961, -14.90920654474416907, 63.93529411764704662 ) ) ;
#8035=DIRECTION ( 'NONE',  ( -3.413470714839332458E-33, 1.190614954331866791E-16, -1.000000000000000000 ) ) ;
#8037=VECTOR ( 'NONE', #47665, 1000.000000000000000 ) ;
#8041=CARTESIAN_POINT ( 'NONE',  ( -24.72409385541305582, -14.80920654474424225, 70.97647058823527288 ) ) ;
#8043=ORIENTED_EDGE ( 'NONE', *, *, #663, .T. ) ;
#8044=CARTESIAN_POINT ( 'NONE',  ( -50.42609385541305755, -14.90920654474413887, 60.01764705882352047 ) ) ;
#8049=CARTESIAN_POINT ( 'NONE',  ( -24.72409385541305582, -14.80920654474419962, 66.05294117647058272 ) ) ;
#8055=CARTESIAN_POINT ( 'NONE',  ( -50.42409385541305511, -14.80920654474410725, 74.99999999999998579 ) ) ;
#8056=LINE ( 'NONE', #38053, #36785 ) ;
#8060=ORIENTED_EDGE ( 'NONE', *, *, #48452, .F. ) ;
#8063=ORIENTED_EDGE ( 'NONE', *, *, #3961, .F. ) ;
#8084=ORIENTED_EDGE ( 'NONE', *, *, #45828, .F. ) ;
#8100=ORIENTED_EDGE ( 'NONE', *, *, #3638, .T. ) ;
#8107=LINE ( 'NONE', #27042, #18950 ) ;
#8150=CARTESIAN_POINT ( 'NONE',  ( -24.72409385541305582, -14.80920654474415699, 62.02941176470587692 ) ) ;
#8156=FACE_OUTER_BOUND ( 'NONE', #22384, .T. ) ;
#8157=AXIS2_PLACEMENT_3D ( 'NONE', #24683, #39688, #31333 ) ;
#8161=EDGE_CURVE ( 'NONE', #8614, #38441, #11666, .T. ) ;
#8166=LINE ( 'NONE', #7432, #34517 ) ;
#8201=ORIENTED_EDGE ( 'NONE', *, *, #44885, .F. ) ;
#8210=CARTESIAN_POINT ( 'NONE',  ( -50.42609385541305755, -14.90920654474423301, 69.97058823529410176 ) ) ;
#8220=CARTESIAN_POINT ( 'NONE',  ( -50.42609385541305755, -14.80920654474421205, 67.05882352941175384 ) ) ;
#8234=DIRECTION ( 'NONE',  ( -2.866981220435666553E-17, 1.000000000000000000, 1.190614954331866791E-16 ) ) ;
#8236=EDGE_LOOP ( 'NONE', ( #17613, #14548, #29950, #5178 ) ) ;
#8268=CARTESIAN_POINT ( 'NONE',  ( -41.16232914953070576, -14.90920654474427565, 73.09411764705880898 ) ) ;
#8283=DIRECTION ( 'NONE',  ( -1.000000000000000000, -2.866981220435666553E-17, 0.000000000000000000 ) ) ;
#8304=LINE ( 'NONE', #16396, #1372 ) ;
#8308=LINE ( 'NONE', #31191, #22907 ) ;
#8335=ORIENTED_EDGE ( 'NONE', *, *, #44079, .F. ) ;
#8392=CARTESIAN_POINT ( 'NONE',  ( -50.42609385541305755, -14.90920654474426499, 72.98823529411762934 ) ) ;
#8404=CARTESIAN_POINT ( 'NONE',  ( -41.41379973776600565, -14.90920654474425433, 71.08235294117645253 ) ) ;
#8415=CARTESIAN_POINT ( 'NONE',  ( -50.42609385541305755, -14.80920654474416764, 63.03529411764704804 ) ) ;
#8471=ORIENTED_EDGE ( 'NONE', *, *, #34691, .F. ) ;
#8531=ORIENTED_EDGE ( 'NONE', *, *, #7106, .F. ) ;
#8552=AXIS2_PLACEMENT_3D ( 'NONE', #32834, #37246, #3296 ) ;
#8564=AXIS2_PLACEMENT_3D ( 'NONE', #43464, #6016, #2801 ) ;
#8584=FACE_OUTER_BOUND ( 'NONE', #38452, .T. ) ;
#8589=VERTEX_POINT ( 'NONE', #39645 ) ;
#8596=LINE ( 'NONE', #4907, #3810 ) ;
#8597=PRODUCT_DEFINITION_FORMATION_WITH_SPECIFIED_SOURCE ( 'ANY', '', #33845, .NOT_KNOWN. ) ;
#8612=DIRECTION ( 'NONE',  ( 1.000000000000000000, 2.866981220435666553E-17, 0.000000000000000000 ) ) ;
#8614=VERTEX_POINT ( 'NONE', #40138 ) ;
#8630=ORIENTED_EDGE ( 'NONE', *, *, #26631, .F. ) ;
#8633=ORIENTED_EDGE ( 'NONE', *, *, #6938, .F. ) ;
#8664=DIRECTION ( 'NONE',  ( 1.000000000000000000, 0.000000000000000000, 0.000000000000000000 ) ) ;
#8671=AXIS2_PLACEMENT_3D ( 'NONE', #32630, #36776, #28694 ) ;
#8720=CARTESIAN_POINT ( 'NONE',  ( -50.42609385541305755, -14.80920654474424225, 70.07647058823528141 ) ) ;
#8732=CARTESIAN_POINT ( 'NONE',  ( -41.53953503188365204, -14.80920654474424225, 70.07647058823528141 ) ) ;
#8745=VECTOR ( 'NONE', #42043, 1000.000000000000000 ) ;
#8791=DIRECTION ( 'NONE',  ( -2.866981220435666553E-17, 1.000000000000000000, 1.190614954331866791E-16 ) ) ;
#8825=ORIENTED_EDGE ( 'NONE', *, *, #48452, .T. ) ;
#8828=EDGE_LOOP ( 'NONE', ( #13933, #28951, #33081, #35298 ) ) ;
#8850=CARTESIAN_POINT ( 'NONE',  ( -41.79100562011894482, -14.80920654474422271, 68.06470588235292496 ) ) ;
#8924=CARTESIAN_POINT ( 'NONE',  ( -43.06159385541306506, -14.80920654474410902, 57.89999999999999147 ) ) ;
#8940=DIRECTION ( 'NONE',  ( 2.866981220435666553E-17, -1.000000000000000000, -1.190614954331866791E-16 ) ) ;
#8961=DIRECTION ( 'NONE',  ( 2.866981220435666553E-17, -1.000000000000000000, -1.190614954331866791E-16 ) ) ;
#8985=EDGE_CURVE ( 'NONE', #454, #26524, #26211, .T. ) ;
#9009=EDGE_CURVE ( 'NONE', #23509, #35946, #15107, .T. ) ;
#9042=ORIENTED_EDGE ( 'NONE', *, *, #15248, .F. ) ;
#9044=CARTESIAN_POINT ( 'NONE',  ( -41.91674091423659121, -14.80920654474410547, 67.05882352941175384 ) ) ;
#9061=DIRECTION ( 'NONE',  ( -1.000000000000000000, -2.866981220435666553E-17, -0.000000000000000000 ) ) ;
#9082=PLANE ( 'NONE',  #11551 ) ;
#9161=AXIS2_PLACEMENT_3D ( 'NONE', #17398, #31701, #9061 ) ;
#9175=CARTESIAN_POINT ( 'NONE',  ( -24.72409385541305582, -14.90920654474425255, 71.98235294117645822 ) ) ;
#9222=ADVANCED_FACE ( 'NONE', ( #24477 ), #35765, .T. ) ;
#9229=LINE ( 'NONE', #23772, #1548 ) ;
#9232=ORIENTED_EDGE ( 'NONE', *, *, #7226, .T. ) ;
#9239=AXIS2_PLACEMENT_3D ( 'NONE', #4433, #15493, #12550 ) ;
#9285=CARTESIAN_POINT ( 'NONE',  ( -41.17556444364835500, -14.80920654474426534, 72.98823529411762934 ) ) ;
#9291=VECTOR ( 'NONE', #35317, 1000.000000000000000 ) ;
#9300=ORIENTED_EDGE ( 'NONE', *, *, #3332, .F. ) ;
#9308=VERTEX_POINT ( 'NONE', #44630 ) ;
#9314=ORIENTED_EDGE ( 'NONE', *, *, #15185, .T. ) ;
#9343=EDGE_CURVE ( 'NONE', #29232, #38441, #37449, .T. ) ;
#9361=ORIENTED_EDGE ( 'NONE', *, *, #1620, .F. ) ;
#9362=CARTESIAN_POINT ( 'NONE',  ( -50.42609385541305755, -14.90920654474422058, 68.06470588235292496 ) ) ;
#9365=ORIENTED_EDGE ( 'NONE', *, *, #1561, .F. ) ;
#9372=VECTOR ( 'NONE', #12601, 1000.000000000000000 ) ;
#9385=CARTESIAN_POINT ( 'NONE',  ( -24.72409385541305582, -14.90920654474428630, 74.09999999999998010 ) ) ;
#9394=EDGE_LOOP ( 'NONE', ( #2721, #26083, #45524, #37326 ) ) ;
#9395=ORIENTED_EDGE ( 'NONE', *, *, #11731, .T. ) ;
#9403=AXIS2_PLACEMENT_3D ( 'NONE', #43365, #31543, #35696 ) ;
#9409=AXIS2_PLACEMENT_3D ( 'NONE', #32614, #6027, #13639 ) ;
#9418=CARTESIAN_POINT ( 'NONE',  ( -50.42609385541305755, -14.80920654474423159, 69.07058823529411029 ) ) ;
#9422=FACE_OUTER_BOUND ( 'NONE', #32956, .T. ) ;
#9461=ORIENTED_EDGE ( 'NONE', *, *, #23526, .T. ) ;
#9472=ORIENTED_EDGE ( 'NONE', *, *, #33306, .F. ) ;
#9488=VECTOR ( 'NONE', #40551, 1000.000000000000114 ) ;
#9510=ORIENTED_EDGE ( 'NONE', *, *, #22788, .F. ) ;
#9536=AXIS2_PLACEMENT_3D ( 'NONE', #24782, #9990, #28223 ) ;
#9561=LINE ( 'NONE', #39579, #37664 ) ;
#9570=EDGE_CURVE ( 'NONE', #9308, #30495, #37866, .T. ) ;
#9591=ORIENTED_EDGE ( 'NONE', *, *, #28024, .T. ) ;
#9601=CARTESIAN_POINT ( 'NONE',  ( -41.04982914953070861, -14.90920654474427565, 73.99411764705880046 ) ) ;
#9627=ORIENTED_EDGE ( 'NONE', *, *, #11815, .T. ) ;
#9646=ORIENTED_EDGE ( 'NONE', *, *, #31562, .T. ) ;
#9669=FACE_OUTER_BOUND ( 'NONE', #15978, .T. ) ;
#9673=CARTESIAN_POINT ( 'NONE',  ( -24.72409385541305582, -14.80920654474418896, 65.94705882352940307 ) ) ;
#9692=CARTESIAN_POINT ( 'NONE',  ( -24.72409385541305582, -14.90920654474414775, 61.02352941176469869 ) ) ;
#9705=CARTESIAN_POINT ( 'NONE',  ( -50.42609385541305755, -14.80920654474423159, 69.97058823529410176 ) ) ;
#9725=EDGE_LOOP ( 'NONE', ( #11244, #45278, #14368, #35975 ) ) ;
#9741=CARTESIAN_POINT ( 'NONE',  ( -50.42409385541305511, -14.80920654474410725, 74.99999999999998579 ) ) ;
#9765=EDGE_CURVE ( 'NONE', #26524, #33229, #46231, .T. ) ;
#9796=DIRECTION ( 'NONE',  ( -2.866981220435666553E-17, 1.000000000000000000, 1.190614954331866791E-16 ) ) ;
#9806=DIRECTION ( 'NONE',  ( 1.000000000000000000, 2.866981220435666553E-17, 0.000000000000000000 ) ) ;
#9828=VECTOR ( 'NONE', #37956, 1000.000000000000000 ) ;
#9834=DIRECTION ( 'NONE',  ( 1.000000000000000000, 2.866981220435666553E-17, 0.000000000000000000 ) ) ;
#9848=DIRECTION ( 'NONE',  ( -3.413470714839332458E-33, 1.190614954331866791E-16, -1.000000000000000000 ) ) ;
#9871=FACE_OUTER_BOUND ( 'NONE', #39643, .T. ) ;
#9903=LINE ( 'NONE', #2263, #5448 ) ;
#9904=CARTESIAN_POINT ( 'NONE',  ( -24.72409385541305582, -14.80920654474414810, 61.92352941176469727 ) ) ;
#9912=ORIENTED_EDGE ( 'NONE', *, *, #37031, .T. ) ;
#9927=ORIENTED_EDGE ( 'NONE', *, *, #3692, .T. ) ;
#9929=LINE ( 'NONE', #40213, #16406 ) ;
#9990=DIRECTION ( 'NONE',  ( 3.413470714839332458E-33, -1.190614954331866791E-16, 1.000000000000000000 ) ) ;
#10008=EDGE_CURVE ( 'NONE', #7399, #26571, #13168, .T. ) ;
#10012=VERTEX_POINT ( 'NONE', #13418 ) ;
#10055=CARTESIAN_POINT ( 'NONE',  ( -50.42609385541305755, -14.90920654474424367, 70.97647058823527288 ) ) ;
#10069=DIRECTION ( 'NONE',  ( -1.000000000000000000, -2.866981220435666553E-17, 0.000000000000000000 ) ) ;
#10106=AXIS2_PLACEMENT_3D ( 'NONE', #36821, #22075, #21826 ) ;
#10119=VERTEX_POINT ( 'NONE', #7767 ) ;
#10129=ORIENTED_EDGE ( 'NONE', *, *, #41438, .T. ) ;
#10166=DIRECTION ( 'NONE',  ( -2.866981220435666553E-17, 1.000000000000000000, 1.190614954331866791E-16 ) ) ;
#10167=CARTESIAN_POINT ( 'NONE',  ( -47.17409385541305511, -15.81020654474410847, 70.50000000000000000 ) ) ;
#10207=DIRECTION ( 'NONE',  ( -0.1240347345892086062, 1.145860353393066553E-16, -0.9922778767136676281 ) ) ;
#10215=VECTOR ( 'NONE', #46741, 1000.000000000000000 ) ;
#10220=EDGE_CURVE ( 'NONE', #37693, #4839, #38249, .T. ) ;
#10227=LINE ( 'NONE', #13405, #17214 ) ;
#10233=VECTOR ( 'NONE', #26081, 1000.000000000000000 ) ;
#10286=ADVANCED_FACE ( 'NONE', ( #31621 ), #1815, .T. ) ;
#10309=AXIS2_PLACEMENT_3D ( 'NONE', #39284, #8283, #23301 ) ;
#10335=CARTESIAN_POINT ( 'NONE',  ( -40.92409385541305511, -14.80920654474410725, 74.99999999999998579 ) ) ;
#10337=ORIENTED_EDGE ( 'NONE', *, *, #37031, .F. ) ;
#10363=ORIENTED_EDGE ( 'NONE', *, *, #10008, .T. ) ;
#10367=DIRECTION ( 'NONE',  ( -0.1240347345892086200, 1.145860353393066553E-16, -0.9922778767136676281 ) ) ;
#10368=CARTESIAN_POINT ( 'NONE',  ( -50.42609385541305755, -14.90920654474425433, 71.08235294117645253 ) ) ;
#10376=EDGE_CURVE ( 'NONE', #10119, #7399, #10657, .T. ) ;
#10394=CARTESIAN_POINT ( 'NONE',  ( -42.68438797306012589, -14.80920654474413745, 60.91764705882351905 ) ) ;
#10395=DIRECTION ( 'NONE',  ( 3.413470714839332458E-33, -1.190614954331866791E-16, 1.000000000000000000 ) ) ;
#10397=CARTESIAN_POINT ( 'NONE',  ( -24.72409385541305582, -14.80920654474414810, 61.02352941176469869 ) ) ;
#10404=ORIENTED_EDGE ( 'NONE', *, *, #27043, .F. ) ;
#10409=DIRECTION ( 'NONE',  ( -2.866981220435666553E-17, 1.000000000000000000, 1.190614954331866791E-16 ) ) ;
#10420=CARTESIAN_POINT ( 'NONE',  ( -50.42609385541305755, -14.80920654474425291, 71.98235294117645822 ) ) ;
#10441=ORIENTED_EDGE ( 'NONE', *, *, #23275, .T. ) ;
#10449=DIRECTION ( 'NONE',  ( 2.866981220435666553E-17, -1.000000000000000000, -1.190614954331866791E-16 ) ) ;
#10459=DIRECTION ( 'NONE',  ( 2.866981220435666553E-17, -1.000000000000000000, -1.190614954331866791E-16 ) ) ;
#10476=DIRECTION ( 'NONE',  ( 1.000000000000000000, 2.866981220435666553E-17, 0.000000000000000000 ) ) ;
#10495=EDGE_CURVE ( 'NONE', #7399, #46865, #7707, .T. ) ;
#10499=ADVANCED_FACE ( 'NONE', ( #37960, #41911, #26169 ), #790, .F. ) ;
#10518=CARTESIAN_POINT ( 'NONE',  ( -40.92409385541305511, -14.80920654474410725, 74.99999999999998579 ) ) ;
#10523=LINE ( 'NONE', #17411, #7041 ) ;
#10544=VERTEX_POINT ( 'NONE', #34022 ) ;
#10550=CARTESIAN_POINT ( 'NONE',  ( -50.42609385541305755, -14.90920654474417972, 64.04117647058822627 ) ) ;
#10593=AXIS2_PLACEMENT_3D ( 'NONE', #7084, #430, #6829 ) ;
#10657=LINE ( 'NONE', #40218, #16523 ) ;
#10659=ORIENTED_EDGE ( 'NONE', *, *, #13550, .T. ) ;
#10677=ORIENTED_EDGE ( 'NONE', *, *, #47257, .T. ) ;
#10702=ORIENTED_EDGE ( 'NONE', *, *, #48245, .F. ) ;
#10704=CARTESIAN_POINT ( 'NONE',  ( -50.42609385541305755, -14.90920654474424367, 70.07647058823528141 ) ) ;
#10721=VECTOR ( 'NONE', #7108, 1000.000000000000000 ) ;
#10723=VERTEX_POINT ( 'NONE', #37101 ) ;
#10740=ORIENTED_EDGE ( 'NONE', *, *, #38809, .F. ) ;
#10757=DIRECTION ( 'NONE',  ( -0.1240347345892086200, 1.145860353393066553E-16, -0.9922778767136676281 ) ) ;
#10776=ORIENTED_EDGE ( 'NONE', *, *, #32893, .F. ) ;
#10794=ORIENTED_EDGE ( 'NONE', *, *, #22788, .T. ) ;
#10823=LINE ( 'NONE', #44825, #12481 ) ;
#10833=ORIENTED_EDGE ( 'NONE', *, *, #27009, .T. ) ;
#10839=VECTOR ( 'NONE', #4458, 1000.000000000000000 ) ;
#10846=ORIENTED_EDGE ( 'NONE', *, *, #36443, .F. ) ;
#10898=ORIENTED_EDGE ( 'NONE', *, *, #33515, .T. ) ;
#10904=VECTOR ( 'NONE', #6634, 1000.000000000000114 ) ;
#10907=VECTOR ( 'NONE', #37954, 1000.000000000000000 ) ;
#10933=LINE ( 'NONE', #25953, #43584 ) ;
#10950=ORIENTED_EDGE ( 'NONE', *, *, #6938, .T. ) ;
#10996=LINE ( 'NONE', #6811, #44667 ) ;
#11021=CARTESIAN_POINT ( 'NONE',  ( -24.72409385541305582, -14.80920654474417830, 64.04117647058822627 ) ) ;
#11030=CARTESIAN_POINT ( 'NONE',  ( -50.42609385541305755, -14.80920654474418008, 64.04117647058822627 ) ) ;
#11031=FACE_OUTER_BOUND ( 'NONE', #570, .T. ) ;
#11079=AXIS2_PLACEMENT_3D ( 'NONE', #48224, #9848, #6147 ) ;
#11084=CARTESIAN_POINT ( 'NONE',  ( -24.72409385541305582, -14.90920654474410512, 56.99999999999998579 ) ) ;
#11091=FACE_OUTER_BOUND ( 'NONE', #5572, .T. ) ;
#11106=CARTESIAN_POINT ( 'NONE',  ( -24.72409385541305582, -15.80920654474410725, 65.99999999999998579 ) ) ;
#11133=DIRECTION ( 'NONE',  ( -1.000000000000000000, -2.866981220435666553E-17, -0.000000000000000000 ) ) ;
#11140=LINE ( 'NONE', #6956, #47845 ) ;
#11157=CARTESIAN_POINT ( 'NONE',  ( -50.42609385541305755, -14.90920654474427565, 73.99411764705880046 ) ) ;
#11193=CARTESIAN_POINT ( 'NONE',  ( -41.17556444364835500, -14.90920654474426499, 72.98823529411762934 ) ) ;
#11206=EDGE_CURVE ( 'NONE', #17004, #18610, #37782, .T. ) ;
#11232=VERTEX_POINT ( 'NONE', #30905 ) ;
#11244=ORIENTED_EDGE ( 'NONE', *, *, #347, .F. ) ;
#11245=DIRECTION ( 'NONE',  ( -1.000000000000000000, -2.866981220435666553E-17, -0.000000000000000000 ) ) ;
#11250=ORIENTED_EDGE ( 'NONE', *, *, #31095, .T. ) ;
#11261=DIRECTION ( 'NONE',  ( -3.413470714839332458E-33, 1.190614954331866791E-16, -1.000000000000000000 ) ) ;
#11309=AXIS2_PLACEMENT_3D ( 'NONE', #12618, #17011, #31578 ) ;
#11312=DIRECTION ( 'NONE',  ( -2.866981220435666553E-17, 1.000000000000000000, 1.190614954331866791E-16 ) ) ;
#11320=ORIENTED_EDGE ( 'NONE', *, *, #3638, .F. ) ;
#11349=DIRECTION ( 'NONE',  ( -2.866981220435666553E-17, 1.000000000000000000, 1.190614954331866791E-16 ) ) ;
#11380=FACE_OUTER_BOUND ( 'NONE', #38894, .T. ) ;
#11414=CARTESIAN_POINT ( 'NONE',  ( -50.42609385541305755, -14.90920654474416907, 63.03529411764704804 ) ) ;
#11434=VERTEX_POINT ( 'NONE', #44646 ) ;
#11455=ORIENTED_EDGE ( 'NONE', *, *, #432, .T. ) ;
#11473=ORIENTED_EDGE ( 'NONE', *, *, #27484, .T. ) ;
#11491=LINE ( 'NONE', #41285, #555 ) ;
#11509=AXIS2_PLACEMENT_3D ( 'NONE', #6657, #40869, #22406 ) ;
#11513=CARTESIAN_POINT ( 'NONE',  ( -50.42609385541305755, -14.80920654474411613, 58.00588235294116402 ) ) ;
#11527=EDGE_CURVE ( 'NONE', #18661, #18610, #44902, .T. ) ;
#11540=ORIENTED_EDGE ( 'NONE', *, *, #18323, .T. ) ;
#11551=AXIS2_PLACEMENT_3D ( 'NONE', #16683, #28269, #31723 ) ;
#11569=ORIENTED_EDGE ( 'NONE', *, *, #15248, .T. ) ;
#11594=DIRECTION ( 'NONE',  ( 1.000000000000000000, 2.866981220435666553E-17, 0.000000000000000000 ) ) ;
#11599=CARTESIAN_POINT ( 'NONE',  ( -24.72409385541305582, -14.80920654474421028, 67.05882352941175384 ) ) ;
#11614=LINE ( 'NONE', #23434, #45243 ) ;
#11621=LINE ( 'NONE', #41663, #45270 ) ;
#11623=CARTESIAN_POINT ( 'NONE',  ( -50.42409385541305511, -15.80920654474410725, 65.99999999999998579 ) ) ;
#11657=FACE_OUTER_BOUND ( 'NONE', #19495, .T. ) ;
#11666=LINE ( 'NONE', #34546, #18028 ) ;
#11675=CARTESIAN_POINT ( 'NONE',  ( -50.42609385541305755, -14.80920654474420139, 66.95294117647057419 ) ) ;
#11676=ADVANCED_FACE ( 'NONE', ( #46820 ), #24423, .T. ) ;
#11731=EDGE_CURVE ( 'NONE', #45977, #18743, #5939, .T. ) ;
#11746=ADVANCED_FACE ( 'NONE', ( #36203 ), #2485, .T. ) ;
#11762=VECTOR ( 'NONE', #15652, 1000.000000000000000 ) ;
#11815=EDGE_CURVE ( 'NONE', #13312, #15919, #33968, .T. ) ;
#11823=CARTESIAN_POINT ( 'NONE',  ( -24.72409385541305582, -14.80920654474411613, 58.90588235294116970 ) ) ;
#11834=ORIENTED_EDGE ( 'NONE', *, *, #6759, .F. ) ;
#11837=CARTESIAN_POINT ( 'NONE',  ( -24.72409385541305582, -14.90920654474419038, 65.04705882352939739 ) ) ;
#11876=EDGE_CURVE ( 'NONE', #47620, #36414, #7157, .T. ) ;
#11892=DIRECTION ( 'NONE',  ( 3.413470714839332458E-33, -1.190614954331866791E-16, 1.000000000000000000 ) ) ;
#11906=DIRECTION ( 'NONE',  ( -3.413470714839332458E-33, 1.190614954331866791E-16, -1.000000000000000000 ) ) ;
#11908=CARTESIAN_POINT ( 'NONE',  ( -41.28806444364835215, -14.80920654474410725, 72.08823529411763786 ) ) ;
#11974=VERTEX_POINT ( 'NONE', #45808 ) ;
#11991=LINE ( 'NONE', #660, #27921 ) ;
#12009=LINE ( 'NONE', #42774, #8745 ) ;
#12016=VERTEX_POINT ( 'NONE', #47251 ) ;
#12041=CARTESIAN_POINT ( 'NONE',  ( -41.92997620835424044, -14.90920654474420104, 66.95294117647057419 ) ) ;
#12078=DIRECTION ( 'NONE',  ( -0.1240347345892086200, 1.145860353393066553E-16, -0.9922778767136676281 ) ) ;
#12087=DIRECTION ( 'NONE',  ( 2.866981220435666553E-17, -1.000000000000000000, -1.190614954331866791E-16 ) ) ;
#12089=PLANE ( 'NONE',  #19525 ) ;
#12092=ORIENTED_EDGE ( 'NONE', *, *, #29570, .T. ) ;
#12108=LINE ( 'NONE', #27124, #13005 ) ;
#12130=EDGE_LOOP ( 'NONE', ( #29730, #40693, #37273, #3711 ) ) ;
#12150=ADVANCED_FACE ( 'NONE', ( #42469 ), #23274, .F. ) ;
#12197=CARTESIAN_POINT ( 'NONE',  ( -50.42609385541305755, -14.90920654474428630, 74.09999999999998010 ) ) ;
#12228=VERTEX_POINT ( 'NONE', #27922 ) ;
#12234=DIRECTION ( 'NONE',  ( 2.866981220435666553E-17, -1.000000000000000000, -1.190614954331866791E-16 ) ) ;
#12244=AXIS2_PLACEMENT_3D ( 'NONE', #13361, #16813, #32573 ) ;
#12246=CARTESIAN_POINT ( 'NONE',  ( -50.42609385541305755, -14.80920654474422271, 68.06470588235292496 ) ) ;
#12247=EDGE_LOOP ( 'NONE', ( #35853, #36976, #45268, #25438 ) ) ;
#12260=CARTESIAN_POINT ( 'NONE',  ( -44.67409385541304800, -14.80920654474410725, 70.50000000000000000 ) ) ;
#12270=LINE ( 'NONE', #5630, #10215 ) ;
#12284=ORIENTED_EDGE ( 'NONE', *, *, #46588, .F. ) ;
#12330=EDGE_CURVE ( 'NONE', #30065, #19883, #20299, .T. ) ;
#12350=ORIENTED_EDGE ( 'NONE', *, *, #34691, .T. ) ;
#12351=VECTOR ( 'NONE', #34863, 1000.000000000000114 ) ;
#12359=CARTESIAN_POINT ( 'NONE',  ( -42.54541738482483026, -14.80920654474415699, 62.02941176470587692 ) ) ;
#12392=VECTOR ( 'NONE', #11906, 1000.000000000000000 ) ;
#12404=PLANE ( 'NONE',  #42622 ) ;
#12414=VECTOR ( 'NONE', #21641, 1000.000000000000000 ) ;
#12421=VECTOR ( 'NONE', #2862, 1000.000000000000000 ) ;
#12441=DIRECTION ( 'NONE',  ( 1.000000000000000000, 2.866981220435666553E-17, 0.000000000000000000 ) ) ;
#12454=EDGE_CURVE ( 'NONE', #26524, #37287, #18276, .T. ) ;
#12481=VECTOR ( 'NONE', #37147, 1000.000000000000114 ) ;
#12531=DIRECTION ( 'NONE',  ( 2.866981220435666553E-17, -1.000000000000000000, -1.190614954331866791E-16 ) ) ;
#12543=LINE ( 'NONE', #31258, #3919 ) ;
#12546=VECTOR ( 'NONE', #21155, 1000.000000000000000 ) ;
#12550=DIRECTION ( 'NONE',  ( -2.866981220435666553E-17, 1.000000000000000000, 1.190614954331866791E-16 ) ) ;
#12551=ORIENTED_EDGE ( 'NONE', *, *, #27819, .T. ) ;
#12557=ORIENTED_EDGE ( 'NONE', *, *, #3390, .F. ) ;
#12560=EDGE_CURVE ( 'NONE', #17265, #17004, #41190, .T. ) ;
#12584=ORIENTED_EDGE ( 'NONE', *, *, #27608, .F. ) ;
#12600=ORIENTED_EDGE ( 'NONE', *, *, #30501, .T. ) ;
#12601=DIRECTION ( 'NONE',  ( -2.866981220435666553E-17, 1.000000000000000000, 1.190614954331866791E-16 ) ) ;
#12603=CLOSED_SHELL ( 'NONE', ( #7942, #3398, #6308, #44340, #32890, #34737, #19150, #10499, #17965, #26228, #13250, #46307, #5210, #32344, #32139, #39474, #18821, #44812, #17304, #33813, #17086, #3977, #26468, #37968, #3255, #5267, #13327, #22438, #35948, #9222, #18316, #20053, #41053, #40488, #43718, #29344, #47476, #42224, #14680, #7946, #44526, #28777, #43002, #15577, #30564, #19573, #44740, #25041, #40287, #11676, #36193, #46999, #17844, #44714, #12150, #2502, #19496, #4555, #24387, #22861, #31568, #16689, #29404, #11746, #46084, #6054, #2077, #38549, #30902, #30771, #46782, #41978, #25491, #10286, #14201, #19827, #20591, #12663, #33709, #33713 ) ) ;
#12618=CARTESIAN_POINT ( 'NONE',  ( -50.42609385541305755, -14.90920654474413887, 60.01764705882352047 ) ) ;
#12629=DIRECTION ( 'NONE',  ( 1.000000000000000000, 0.000000000000000000, 0.000000000000000000 ) ) ;
#12663=ADVANCED_FACE ( 'NONE', ( #2003 ), #16998, .F. ) ;
#12710=DIRECTION ( 'NONE',  ( -2.866981220435666553E-17, 1.000000000000000000, 1.190614954331866791E-16 ) ) ;
#12741=LINE ( 'NONE', #1164, #815 ) ;
#12762=ORIENTED_EDGE ( 'NONE', *, *, #19653, .F. ) ;
#12788=PLANE ( 'NONE',  #9239 ) ;
#12819=DIRECTION ( 'NONE',  ( -2.866981220435666553E-17, 1.000000000000000000, 1.190614954331866791E-16 ) ) ;
#12863=DIRECTION ( 'NONE',  ( 1.000000000000000000, 2.866981220435666553E-17, 0.000000000000000000 ) ) ;
#12897=DIRECTION ( 'NONE',  ( -3.413470714839332458E-33, 1.190614954331866791E-16, -1.000000000000000000 ) ) ;
#12901=VERTEX_POINT ( 'NONE', #529 ) ;
#12927=VERTEX_POINT ( 'NONE', #8404 ) ;
#12930=ORIENTED_EDGE ( 'NONE', *, *, #3544, .F. ) ;
#12944=VECTOR ( 'NONE', #20847, 1000.000000000000000 ) ;
#12970=ORIENTED_EDGE ( 'NONE', *, *, #45087, .T. ) ;
#12978=PRODUCT_DEFINITION_CONTEXT ( 'detailed design', #46687, 'design' ) ;
#12988=EDGE_CURVE ( 'NONE', #13624, #46626, #31056, .T. ) ;
#13002=DIRECTION ( 'NONE',  ( 2.866981220435666553E-17, -1.000000000000000000, -1.190614954331866791E-16 ) ) ;
#13005=VECTOR ( 'NONE', #4004, 1000.000000000000000 ) ;
#13079=ORIENTED_EDGE ( 'NONE', *, *, #1212, .F. ) ;
#13081=LINE ( 'NONE', #9418, #39336 ) ;
#13106=ORIENTED_EDGE ( 'NONE', *, *, #19160, .T. ) ;
#13109=VECTOR ( 'NONE', #24735, 1000.000000000000000 ) ;
#13115=DIRECTION ( 'NONE',  ( 2.866981220435666553E-17, -1.000000000000000000, -1.190614954331866791E-16 ) ) ;
#13142=EDGE_CURVE ( 'NONE', #21061, #20803, #14472, .T. ) ;
#13162=ORIENTED_EDGE ( 'NONE', *, *, #39849, .F. ) ;
#13168=LINE ( 'NONE', #1626, #41714 ) ;
#13174=AXIS2_PLACEMENT_3D ( 'NONE', #5734, #6681, #17015 ) ;
#13175=PLANE ( 'NONE',  #9536 ) ;
#13182=CARTESIAN_POINT ( 'NONE',  ( -24.72409385541305582, -14.90920654474416729, 63.03529411764704804 ) ) ;
#13184=ORIENTED_EDGE ( 'NONE', *, *, #48245, .T. ) ;
#13188=LINE ( 'NONE', #39559, #12944 ) ;
#13222=DIRECTION ( 'NONE',  ( 3.413470714839332458E-33, -1.190614954331866791E-16, 1.000000000000000000 ) ) ;
#13235=DIRECTION ( 'NONE',  ( 1.000000000000000000, 2.866981220435666553E-17, 0.000000000000000000 ) ) ;
#13246=ORIENTED_EDGE ( 'NONE', *, *, #5938, .F. ) ;
#13249=DIRECTION ( 'NONE',  ( 2.866981220435666553E-17, -1.000000000000000000, -1.190614954331866791E-16 ) ) ;
#13250=ADVANCED_FACE ( 'NONE', ( #29784 ), #38126, .T. ) ;
#13299=VECTOR ( 'NONE', #47940, 1000.000000000000114 ) ;
#13307=DIRECTION ( 'NONE',  ( 2.866981220435666553E-17, -1.000000000000000000, -1.190614954331866791E-16 ) ) ;
#13312=VERTEX_POINT ( 'NONE', #12041 ) ;
#13327=ADVANCED_FACE ( 'NONE', ( #16193 ), #1430, .F. ) ;
#13329=LINE ( 'NONE', #9673, #23738 ) ;
#13340=DIRECTION ( 'NONE',  ( 2.866981220435666553E-17, -1.000000000000000000, -1.190614954331866791E-16 ) ) ;
#13341=ORIENTED_EDGE ( 'NONE', *, *, #33515, .F. ) ;
#13350=VECTOR ( 'NONE', #34925, 1000.000000000000000 ) ;
#13361=CARTESIAN_POINT ( 'NONE',  ( -50.42609385541305755, -14.80920654474421205, 67.95882352941174531 ) ) ;
#13363=CARTESIAN_POINT ( 'NONE',  ( -47.17409385541305511, -14.80920654474410725, 70.50000000000000000 ) ) ;
#13381=CARTESIAN_POINT ( 'NONE',  ( -24.72409385541305582, -14.80920654474415699, 62.92941176470587550 ) ) ;
#13391=ORIENTED_EDGE ( 'NONE', *, *, #37268, .T. ) ;
#13405=CARTESIAN_POINT ( 'NONE',  ( -24.72409385541305582, -14.80920654474416764, 63.03529411764704804 ) ) ;
#13418=CARTESIAN_POINT ( 'NONE',  ( -24.72409385541305582, -14.90920654474421170, 67.95882352941174531 ) ) ;
#13460=UNCERTAINTY_MEASURE_WITH_UNIT (LENGTH_MEASURE( 1.000000000000000082E-05 ), #5412, 'distance_accuracy_value', 'NONE');
#13507=ORIENTED_EDGE ( 'NONE', *, *, #40077, .T. ) ;
#13544=ORIENTED_EDGE ( 'NONE', *, *, #34007, .T. ) ;
#13550=EDGE_CURVE ( 'NONE', #19851, #47529, #21843, .T. ) ;
#13558=CARTESIAN_POINT ( 'NONE',  ( -50.42609385541305755, -14.90920654474419038, 65.94705882352940307 ) ) ;
#13571=ORIENTED_EDGE ( 'NONE', *, *, #6759, .T. ) ;
#13572=CARTESIAN_POINT ( 'NONE',  ( -50.42609385541305755, -14.90920654474425433, 71.08235294117645253 ) ) ;
#13586=DIRECTION ( 'NONE',  ( 3.413470714839332458E-33, -1.190614954331866791E-16, 1.000000000000000000 ) ) ;
#13599=PLANE ( 'NONE',  #43292 ) ;
#13622=LINE ( 'NONE', #13381, #32979 ) ;
#13624=VERTEX_POINT ( 'NONE', #30469 ) ;
#13628=ORIENTED_EDGE ( 'NONE', *, *, #3961, .T. ) ;
#13639=DIRECTION ( 'NONE',  ( 1.000000000000000000, 0.000000000000000000, 0.000000000000000000 ) ) ;
#13653=DIRECTION ( 'NONE',  ( 1.000000000000000000, 2.866981220435666553E-17, 0.000000000000000000 ) ) ;
#13654=ORIENTED_EDGE ( 'NONE', *, *, #2661, .T. ) ;
#13664=VECTOR ( 'NONE', #25229, 1000.000000000000000 ) ;
#13665=CARTESIAN_POINT ( 'NONE',  ( -50.42609385541305755, -14.80920654474428666, 74.09999999999998010 ) ) ;
#13669=EDGE_CURVE ( 'NONE', #22665, #29528, #38299, .T. ) ;
#13723=ORIENTED_EDGE ( 'NONE', *, *, #31158, .T. ) ;
#13734=LINE ( 'NONE', #13971, #37525 ) ;
#13819=ORIENTED_EDGE ( 'NONE', *, *, #33522, .F. ) ;
#13893=EDGE_CURVE ( 'NONE', #42385, #18335, #38187, .T. ) ;
#13901=VECTOR ( 'NONE', #19486, 1000.000000000000000 ) ;
#13927=EDGE_CURVE ( 'NONE', #41894, #39596, #45617, .T. ) ;
#13933=ORIENTED_EDGE ( 'NONE', *, *, #14015, .T. ) ;
#13942=FACE_OUTER_BOUND ( 'NONE', #23847, .T. ) ;
#13945=AXIS2_PLACEMENT_3D ( 'NONE', #24463, #13340, #39468 ) ;
#13959=DIRECTION ( 'NONE',  ( -3.413470714839332458E-33, 1.190614954331866791E-16, -1.000000000000000000 ) ) ;
#13970=AXIS2_PLACEMENT_3D ( 'NONE', #18240, #25408, #2744 ) ;
#13971=CARTESIAN_POINT ( 'NONE',  ( -50.42609385541305755, -14.90920654474419038, 65.04705882352939739 ) ) ;
#13984=CARTESIAN_POINT ( 'NONE',  ( -24.72409385541305582, -14.80920654474427423, 73.09411764705880898 ) ) ;
#14002=CARTESIAN_POINT ( 'NONE',  ( -24.72409385541305582, -14.90920654474423124, 69.97058823529410176 ) ) ;
#14009=ORIENTED_EDGE ( 'NONE', *, *, #8985, .F. ) ;
#14015=EDGE_CURVE ( 'NONE', #18357, #2135, #32034, .T. ) ;
#14071=CARTESIAN_POINT ( 'NONE',  ( -50.42409385541305511, -14.80920654474410547, 56.99999999999998579 ) ) ;
#14082=EDGE_CURVE ( 'NONE', #6974, #8589, #1252, .T. ) ;
#14087=CARTESIAN_POINT ( 'NONE',  ( -42.41905675134066200, -14.90920654474417972, 63.04029683257916616 ) ) ;
#14088=ORIENTED_EDGE ( 'NONE', *, *, #25612, .F. ) ;
#14092=ORIENTED_EDGE ( 'NONE', *, *, #7783, .T. ) ;
#14102=VECTOR ( 'NONE', #24613, 1000.000000000000000 ) ;
#14107=LINE ( 'NONE', #18544, #13664 ) ;
#14124=FACE_OUTER_BOUND ( 'NONE', #27016, .T. ) ;
#14152=ORIENTED_EDGE ( 'NONE', *, *, #47238, .T. ) ;
#14193=DIRECTION ( 'NONE',  ( -2.866981220435666553E-17, 1.000000000000000000, 1.190614954331866791E-16 ) ) ;
#14201=ADVANCED_FACE ( 'NONE', ( #14480 ), #48486, .F. ) ;
#14204=PLANE ( 'NONE',  #16649 ) ;
#14209=ORIENTED_EDGE ( 'NONE', *, *, #19149, .T. ) ;
#14224=EDGE_CURVE ( 'NONE', #16499, #45977, #4188, .T. ) ;
#14230=DIRECTION ( 'NONE',  ( -2.866981220435666553E-17, 1.000000000000000000, 1.190614954331866791E-16 ) ) ;
#14232=CARTESIAN_POINT ( 'NONE',  ( -40.92409385541305511, -14.80920654474410725, 74.99999999999998579 ) ) ;
#14233=ORIENTED_EDGE ( 'NONE', *, *, #46363, .F. ) ;
#14266=VECTOR ( 'NONE', #25915, 1000.000000000000000 ) ;
#14295=VERTEX_POINT ( 'NONE', #23375 ) ;
#14300=DIRECTION ( 'NONE',  ( -1.000000000000000000, -2.866981220435666553E-17, 0.000000000000000000 ) ) ;
#14320=ORIENTED_EDGE ( 'NONE', *, *, #42686, .T. ) ;
#14336=CARTESIAN_POINT ( 'NONE',  ( -42.16821150247188399, -14.80920654474418896, 65.04705882352939739 ) ) ;
#14368=ORIENTED_EDGE ( 'NONE', *, *, #28510, .T. ) ;
#14394=CARTESIAN_POINT ( 'NONE',  ( -44.67409385541304800, -15.80920654474410725, 70.50000000000000000 ) ) ;
#14413=ORIENTED_EDGE ( 'NONE', *, *, #38380, .T. ) ;
#14420=CARTESIAN_POINT ( 'NONE',  ( -24.72409385541305582, -14.80920654474419962, 66.95294117647057419 ) ) ;
#14450=ORIENTED_EDGE ( 'NONE', *, *, #23807, .T. ) ;
#14472=LINE ( 'NONE', #2466, #48502 ) ;
#14473=EDGE_CURVE ( 'NONE', #27084, #46946, #36846, .T. ) ;
#14480=FACE_OUTER_BOUND ( 'NONE', #25428, .T. ) ;
#14514=ORIENTED_EDGE ( 'NONE', *, *, #34637, .T. ) ;
#14522=DIRECTION ( 'NONE',  ( -0.1240347345892086200, 1.145860353393066553E-16, -0.9922778767136676281 ) ) ;
#14547=ORIENTED_EDGE ( 'NONE', *, *, #42919, .F. ) ;
#14548=ORIENTED_EDGE ( 'NONE', *, *, #1487, .T. ) ;
#14563=EDGE_LOOP ( 'NONE', ( #5362, #35544, #19797, #42840 ) ) ;
#14571=CARTESIAN_POINT ( 'NONE',  ( -40.92409385541305511, -14.80920654474410725, 74.99999999999998579 ) ) ;
#14580=DIRECTION ( 'NONE',  ( 2.866981220435666553E-17, -1.000000000000000000, -1.190614954331866791E-16 ) ) ;
#14611=EDGE_CURVE ( 'NONE', #1374, #29698, #8304, .T. ) ;
#14639=ORIENTED_EDGE ( 'NONE', *, *, #10008, .F. ) ;
#14646=ORIENTED_EDGE ( 'NONE', *, *, #3727, .T. ) ;
#14680=ADVANCED_FACE ( 'NONE', ( #2996 ), #40198, .F. ) ;
#14705=CARTESIAN_POINT ( 'NONE',  ( -40.92409385541306222, -14.90920654474428630, 74.99999999999998579 ) ) ;
#14721=CARTESIAN_POINT ( 'NONE',  ( -24.72409385541305582, -15.80920654474410725, 65.99999999999998579 ) ) ;
#14727=VECTOR ( 'NONE', #1727, 1000.000000000000000 ) ;
#14738=DIRECTION ( 'NONE',  ( 2.866981220435666553E-17, -1.000000000000000000, -1.190614954331866791E-16 ) ) ;
#14783=PLANE ( 'NONE',  #7451 ) ;
#14799=VECTOR ( 'NONE', #23236, 1000.000000000000000 ) ;
#14814=CARTESIAN_POINT ( 'NONE',  ( -41.41379973776600565, -14.80920654474410725, 71.08235294117645253 ) ) ;
#14815=ORIENTED_EDGE ( 'NONE', *, *, #19160, .F. ) ;
#14851=VECTOR ( 'NONE', #44744, 1000.000000000000000 ) ;
#14875=ORIENTED_EDGE ( 'NONE', *, *, #19882, .F. ) ;
#14909=EDGE_CURVE ( 'NONE', #26571, #24126, #3164, .T. ) ;
#14922=DIRECTION ( 'NONE',  ( 3.413470714839332458E-33, -1.190614954331866791E-16, 1.000000000000000000 ) ) ;
#14925=VERTEX_POINT ( 'NONE', #6863 ) ;
#14939=ORIENTED_EDGE ( 'NONE', *, *, #45087, .F. ) ;
#15022=VERTEX_POINT ( 'NONE', #7611 ) ;
#15030=ORIENTED_EDGE ( 'NONE', *, *, #26750, .F. ) ;
#15041=DIRECTION ( 'NONE',  ( -0.1240347345892086062, 1.145860353393066553E-16, -0.9922778767136676281 ) ) ;
#15046=DIRECTION ( 'NONE',  ( 2.866981220435666553E-17, -1.000000000000000000, -1.190614954331866791E-16 ) ) ;
#15059=VERTEX_POINT ( 'NONE', #15439 ) ;
#15073=CARTESIAN_POINT ( 'NONE',  ( -24.72409385541305582, -14.80920654474417830, 64.94117647058821774 ) ) ;
#15080=ORIENTED_EDGE ( 'NONE', *, *, #4427, .T. ) ;
#15107=LINE ( 'NONE', #11675, #33782 ) ;
#15160=ORIENTED_EDGE ( 'NONE', *, *, #26053, .T. ) ;
#15172=LINE ( 'NONE', #14420, #1944 ) ;
#15174=ORIENTED_EDGE ( 'NONE', *, *, #19799, .T. ) ;
#15185=EDGE_CURVE ( 'NONE', #29482, #17265, #34899, .T. ) ;
#15212=DIRECTION ( 'NONE',  ( -2.866981220435666553E-17, 1.000000000000000000, 1.190614954331866791E-16 ) ) ;
#15232=SHAPE_REPRESENTATION_RELATIONSHIP ( 'NONE' , 'NONE' ,  #41459, #15583 ) ;
#15234=VERTEX_POINT ( 'NONE', #28731 ) ;
#15237=DIRECTION ( 'NONE',  ( 2.866981220435666553E-17, -1.000000000000000000, -1.190614954331866791E-16 ) ) ;
#15248=EDGE_CURVE ( 'NONE', #36768, #46722, #35857, .T. ) ;
#15321=VECTOR ( 'NONE', #7553, 1000.000000000000000 ) ;
#15364=DIRECTION ( 'NONE',  ( -1.000000000000000000, -2.866981220435666553E-17, 0.000000000000000000 ) ) ;
#15369=LINE ( 'NONE', #7044, #45733 ) ;
#15418=ORIENTED_EDGE ( 'NONE', *, *, #2927, .T. ) ;
#15439=CARTESIAN_POINT ( 'NONE',  ( -24.72409385541305582, -14.90920654474413709, 60.91764705882351905 ) ) ;
#15464=AXIS2_PLACEMENT_3D ( 'NONE', #22576, #7568, #45011 ) ;
#15493=DIRECTION ( 'NONE',  ( -3.413470714839332458E-33, 1.190614954331866791E-16, -1.000000000000000000 ) ) ;
#15516=APPLICATION_CONTEXT ( 'automotive_design' ) ;
#15529=AXIS2_PLACEMENT_3D ( 'NONE', #43272, #1892, #27988 ) ;
#15536=VECTOR ( 'NONE', #41696, 1000.000000000000000 ) ;
#15540=VECTOR ( 'NONE', #17940, 1000.000000000000000 ) ;
#15577=ADVANCED_FACE ( 'NONE', ( #19049 ), #40971, .T. ) ;
#15583=ADVANCED_BREP_SHAPE_REPRESENTATION ( '', ( #76, #29031 ), #42412 ) ;
#15602=VECTOR ( 'NONE', #8961, 1000.000000000000000 ) ;
#15630=DIRECTION ( 'NONE',  ( -3.413470714839332458E-33, 1.190614954331866791E-16, -1.000000000000000000 ) ) ;
#15632=ORIENTED_EDGE ( 'NONE', *, *, #26673, .F. ) ;
#15642=CARTESIAN_POINT ( 'NONE',  ( -50.42609385541305755, -14.80920654474415699, 62.92941176470587550 ) ) ;
#15651=ORIENTED_EDGE ( 'NONE', *, *, #38603, .F. ) ;
#15652=DIRECTION ( 'NONE',  ( -3.413470714839332458E-33, 1.190614954331866791E-16, -1.000000000000000000 ) ) ;
#15731=VECTOR ( 'NONE', #22931, 1000.000000000000000 ) ;
#15734=AXIS2_PLACEMENT_3D ( 'NONE', #42615, #27813, #46298 ) ;
#15745=FACE_OUTER_BOUND ( 'NONE', #7872, .T. ) ;
#15749=ORIENTED_EDGE ( 'NONE', *, *, #19653, .T. ) ;
#15750=CARTESIAN_POINT ( 'NONE',  ( -50.42409385541305511, -15.80920654474410725, 74.99999999999998579 ) ) ;
#15784=CARTESIAN_POINT ( 'NONE',  ( -50.42609385541305755, -14.80920654474427600, 73.09411764705880898 ) ) ;
#15811=EDGE_LOOP ( 'NONE', ( #44615, #29176, #13184, #3144 ) ) ;
#15831=ORIENTED_EDGE ( 'NONE', *, *, #44575, .F. ) ;
#15834=ORIENTED_EDGE ( 'NONE', *, *, #27608, .T. ) ;
#15860=CARTESIAN_POINT ( 'NONE',  ( -24.72409385541305582, -15.80920654474410725, 65.99999999999998579 ) ) ;
#15876=VECTOR ( 'NONE', #29059, 1000.000000000000000 ) ;
#15880=LINE ( 'NONE', #4330, #17184 ) ;
#15891=VERTEX_POINT ( 'NONE', #10397 ) ;
#15903=DIRECTION ( 'NONE',  ( 1.000000000000000000, 2.866981220435666553E-17, 0.000000000000000000 ) ) ;
#15919=VERTEX_POINT ( 'NONE', #26372 ) ;
#15924=ORIENTED_EDGE ( 'NONE', *, *, #15185, .F. ) ;
#15978=EDGE_LOOP ( 'NONE', ( #9361, #10794, #42316, #10950 ) ) ;
#16011=ORIENTED_EDGE ( 'NONE', *, *, #32984, .F. ) ;
#16069=CARTESIAN_POINT ( 'NONE',  ( -24.72409385541305582, -14.80920654474415699, 62.92941176470587550 ) ) ;
#16089=CARTESIAN_POINT ( 'NONE',  ( -24.72409385541305582, -14.80920654474421205, 67.95882352941174531 ) ) ;
#16093=EDGE_CURVE ( 'NONE', #19353, #25093, #36355, .T. ) ;
#16094=VECTOR ( 'NONE', #27509, 1000.000000000000000 ) ;
#16121=VERTEX_POINT ( 'NONE', #48175 ) ;
#16130=EDGE_CURVE ( 'NONE', #24230, #6612, #17640, .T. ) ;
#16157=ORIENTED_EDGE ( 'NONE', *, *, #44079, .T. ) ;
#16193=FACE_OUTER_BOUND ( 'NONE', #8236, .T. ) ;
#16256=CARTESIAN_POINT ( 'NONE',  ( -42.04247620835423049, -14.80920654474420139, 66.05294117647058272 ) ) ;
#16290=CARTESIAN_POINT ( 'NONE',  ( -42.68438797306012589, -14.90920654474413709, 60.91764705882351905 ) ) ;
#16293=PLANE ( 'NONE',  #48557 ) ;
#16300=VECTOR ( 'NONE', #35724, 1000.000000000000000 ) ;
#16357=EDGE_LOOP ( 'NONE', ( #17924, #1070, #29299, #46668 ) ) ;
#16368=CARTESIAN_POINT ( 'NONE',  ( -50.42609385541305755, -14.90920654474425433, 71.98235294117645822 ) ) ;
#16371=DIRECTION ( 'NONE',  ( 2.866981220435666553E-17, -1.000000000000000000, -1.190614954331866791E-16 ) ) ;
#16381=VECTOR ( 'NONE', #12441, 1000.000000000000000 ) ;
#16389=CARTESIAN_POINT ( 'NONE',  ( -24.72409385541305582, -14.80920654474414810, 61.02352941176469869 ) ) ;
#16393=EDGE_LOOP ( 'NONE', ( #8201, #14413, #2416, #10846 ) ) ;
#16396=CARTESIAN_POINT ( 'NONE',  ( -24.72409385541305582, -14.80920654474422271, 68.96470588235293064 ) ) ;
#16406=VECTOR ( 'NONE', #15903, 1000.000000000000000 ) ;
#16424=EDGE_CURVE ( 'NONE', #38066, #36768, #39763, .T. ) ;
#16440=ORIENTED_EDGE ( 'NONE', *, *, #43855, .T. ) ;
#16446=DIRECTION ( 'NONE',  ( -0.1240347345892086062, 1.145860353393066553E-16, -0.9922778767136676281 ) ) ;
#16452=ORIENTED_EDGE ( 'NONE', *, *, #26631, .T. ) ;
#16453=EDGE_LOOP ( 'NONE', ( #29588, #6058, #20342, #14875 ) ) ;
#16465=CARTESIAN_POINT ( 'NONE',  ( -24.72409385541305582, -14.80920654474418896, 65.94705882352940307 ) ) ;
#16498=CARTESIAN_POINT ( 'NONE',  ( -41.42703503188364778, -14.80920654474424225, 70.97647058823527288 ) ) ;
#16499=VERTEX_POINT ( 'NONE', #11193 ) ;
#16511=ORIENTED_EDGE ( 'NONE', *, *, #4427, .F. ) ;
#16523=VECTOR ( 'NONE', #24722, 1000.000000000000114 ) ;
#16534=ORIENTED_EDGE ( 'NONE', *, *, #10495, .F. ) ;
#16538=ORIENTED_EDGE ( 'NONE', *, *, #9009, .T. ) ;
#16540=CARTESIAN_POINT ( 'NONE',  ( -24.72409385541305582, -14.80920654474426357, 72.08823529411763786 ) ) ;
#16588=CARTESIAN_POINT ( 'NONE',  ( -24.72409385541305582, -14.90920654474423124, 69.07058823529411029 ) ) ;
#16589=CARTESIAN_POINT ( 'NONE',  ( -24.72409385541305582, -14.80920654474416764, 63.93529411764704662 ) ) ;
#16603=VECTOR ( 'NONE', #48399, 1000.000000000000000 ) ;
#16639=ORIENTED_EDGE ( 'NONE', *, *, #33306, .T. ) ;
#16649=AXIS2_PLACEMENT_3D ( 'NONE', #11513, #41304, #29259 ) ;
#16666=CARTESIAN_POINT ( 'NONE',  ( -40.92409385541305511, -14.80920654474410725, 74.99999999999998579 ) ) ;
#16683=CARTESIAN_POINT ( 'NONE',  ( -50.42609385541305755, -14.80920654474414810, 61.92352941176469727 ) ) ;
#16689=ADVANCED_FACE ( 'NONE', ( #589 ), #42694, .T. ) ;
#16695=EDGE_CURVE ( 'NONE', #17028, #42512, #46383, .T. ) ;
#16700=CARTESIAN_POINT ( 'NONE',  ( -41.30129973776600139, -14.90920654474425433, 71.98235294117645822 ) ) ;
#16745=CARTESIAN_POINT ( 'NONE',  ( -46.92409385541305511, -15.80920654474410725, 61.49999999999999289 ) ) ;
#16772=ORIENTED_EDGE ( 'NONE', *, *, #25612, .T. ) ;
#16813=DIRECTION ( 'NONE',  ( 3.413470714839332458E-33, -1.190614954331866791E-16, 1.000000000000000000 ) ) ;
#16814=CARTESIAN_POINT ( 'NONE',  ( -42.29394679658953038, -14.80920654474410547, 64.04117647058822627 ) ) ;
#16876=FACE_OUTER_BOUND ( 'NONE', #43155, .T. ) ;
#16933=FACE_OUTER_BOUND ( 'NONE', #3984, .T. ) ;
#16935=ORIENTED_EDGE ( 'NONE', *, *, #43855, .F. ) ;
#16946=FILL_AREA_STYLE ('',( #41595 ) ) ;
#16989=ORIENTED_EDGE ( 'NONE', *, *, #38880, .F. ) ;
#16991=LINE ( 'NONE', #32292, #47284 ) ;
#16998=PLANE ( 'NONE',  #35117 ) ;
#17004=VERTEX_POINT ( 'NONE', #41969 ) ;
#17011=DIRECTION ( 'NONE',  ( 2.866981220435666553E-17, -1.000000000000000000, -1.190614954331866791E-16 ) ) ;
#17014=DIRECTION ( 'NONE',  ( 1.000000000000000000, 2.866981220435666553E-17, 0.000000000000000000 ) ) ;
#17015=DIRECTION ( 'NONE',  ( -2.866981220435666553E-17, 1.000000000000000000, 1.190614954331866791E-16 ) ) ;
#17028=VERTEX_POINT ( 'NONE', #39483 ) ;
#17039=CARTESIAN_POINT ( 'NONE',  ( -24.72409385541305582, -14.80920654474424225, 70.07647058823528141 ) ) ;
#17049=VECTOR ( 'NONE', #3214, 1000.000000000000000 ) ;
#17052=FACE_OUTER_BOUND ( 'NONE', #34918, .T. ) ;
#17066=CARTESIAN_POINT ( 'NONE',  ( -24.72409385541305582, -14.90920654474410512, 56.99999999999998579 ) ) ;
#17086=ADVANCED_FACE ( 'NONE', ( #21259 ), #32571, .T. ) ;
#17120=EDGE_CURVE ( 'NONE', #40267, #23016, #6481, .T. ) ;
#17136=CARTESIAN_POINT ( 'NONE',  ( -41.66527032600129132, -14.80920654474423159, 69.07058823529411029 ) ) ;
#17148=CARTESIAN_POINT ( 'NONE',  ( -42.41968209070717677, -14.80920654474416764, 63.03529411764704804 ) ) ;
#17166=LINE ( 'NONE', #28758, #25317 ) ;
#17172=VECTOR ( 'NONE', #39456, 1000.000000000000000 ) ;
#17178=AXIS2_PLACEMENT_3D ( 'NONE', #46619, #39460, #38726 ) ;
#17184=VECTOR ( 'NONE', #15630, 1000.000000000000000 ) ;
#17214=VECTOR ( 'NONE', #25242, 1000.000000000000000 ) ;
#17234=ORIENTED_EDGE ( 'NONE', *, *, #1107, .F. ) ;
#17265=VERTEX_POINT ( 'NONE', #47811 ) ;
#17269=VECTOR ( 'NONE', #23607, 1000.000000000000000 ) ;
#17288=DIRECTION ( 'NONE',  ( 2.866981220435666553E-17, -1.000000000000000000, -1.190614954331866791E-16 ) ) ;
#17304=ADVANCED_FACE ( 'NONE', ( #33250 ), #43898, .F. ) ;
#17320=FACE_OUTER_BOUND ( 'NONE', #29527, .T. ) ;
#17368=AXIS2_PLACEMENT_3D ( 'NONE', #11623, #30358, #48562 ) ;
#17369=LINE ( 'NONE', #32164, #20546 ) ;
#17398=CARTESIAN_POINT ( 'NONE',  ( -50.42609385541305755, -14.90920654474424367, 70.07647058823528141 ) ) ;
#17411=CARTESIAN_POINT ( 'NONE',  ( -24.72409385541305582, -14.90920654474412643, 59.01176470588234224 ) ) ;
#17420=CARTESIAN_POINT ( 'NONE',  ( -24.72409385541305582, -14.90920654474415663, 62.02941176470587692 ) ) ;
#17449=LINE ( 'NONE', #47500, #2150 ) ;
#17455=CARTESIAN_POINT ( 'NONE',  ( -50.42609385541305755, -14.90920654474417972, 64.94117647058821774 ) ) ;
#17490=DIRECTION ( 'NONE',  ( 2.866981220435666553E-17, -1.000000000000000000, -1.190614954331866791E-16 ) ) ;
#17493=CARTESIAN_POINT ( 'NONE',  ( -42.54541738482483026, -14.90920654474415841, 62.02941176470587692 ) ) ;
#17540=PLANE ( 'NONE',  #17675 ) ;
#17562=PLANE ( 'NONE',  #43044 ) ;
#17613=ORIENTED_EDGE ( 'NONE', *, *, #39896, .T. ) ;
#17621=FACE_OUTER_BOUND ( 'NONE', #36554, .T. ) ;
#17627=ORIENTED_EDGE ( 'NONE', *, *, #5059, .F. ) ;
#17640=LINE ( 'NONE', #25524, #36061 ) ;
#17675=AXIS2_PLACEMENT_3D ( 'NONE', #40435, #21499, #29852 ) ;
#17693=LINE ( 'NONE', #36636, #4707 ) ;
#17728=ORIENTED_EDGE ( 'NONE', *, *, #3332, .T. ) ;
#17732=ORIENTED_EDGE ( 'NONE', *, *, #28119, .T. ) ;
#17745=FACE_OUTER_BOUND ( 'NONE', #41232, .T. ) ;
#17746=VERTEX_POINT ( 'NONE', #14705 ) ;
#17798=ORIENTED_EDGE ( 'NONE', *, *, #5712, .F. ) ;
#17809=LINE ( 'NONE', #7498, #48264 ) ;
#17838=EDGE_CURVE ( 'NONE', #41531, #25220, #12270, .T. ) ;
#17844=ADVANCED_FACE ( 'NONE', ( #20640 ), #20397, .T. ) ;
#17859=ORIENTED_EDGE ( 'NONE', *, *, #1915, .F. ) ;
#17874=ORIENTED_EDGE ( 'NONE', *, *, #1916, .T. ) ;
#17876=VECTOR ( 'NONE', #22646, 1000.000000000000114 ) ;
#17877=VECTOR ( 'NONE', #38097, 1000.000000000000000 ) ;
#17893=PLANE ( 'NONE',  #38563 ) ;
#17911=EDGE_CURVE ( 'NONE', #26590, #28413, #10523, .T. ) ;
#17920=CARTESIAN_POINT ( 'NONE',  ( -24.72409385541305582, -14.80920654474413745, 60.91764705882351905 ) ) ;
#17922=ORIENTED_EDGE ( 'NONE', *, *, #663, .F. ) ;
#17924=ORIENTED_EDGE ( 'NONE', *, *, #36392, .F. ) ;
#17940=DIRECTION ( 'NONE',  ( 1.000000000000000000, 2.866981220435666553E-17, 0.000000000000000000 ) ) ;
#17965=ADVANCED_FACE ( 'NONE', ( #29230 ), #44502, .F. ) ;
#18012=DIRECTION ( 'NONE',  ( 1.000000000000000000, 2.866981220435666553E-17, 0.000000000000000000 ) ) ;
#18017=EDGE_CURVE ( 'NONE', #24237, #45073, #653, .T. ) ;
#18028=VECTOR ( 'NONE', #38733, 1000.000000000000000 ) ;
#18063=CARTESIAN_POINT ( 'NONE',  ( -41.55277032600130127, -14.80920654474423159, 69.97058823529410176 ) ) ;
#18086=EDGE_LOOP ( 'NONE', ( #33803, #28253, #9627, #5090 ) ) ;
#18132=CARTESIAN_POINT ( 'NONE',  ( -50.42609385541305755, -14.90920654474411577, 58.00588235294116402 ) ) ;
#18136=DIRECTION ( 'NONE',  ( 3.413470714839332458E-33, -1.190614954331866791E-16, 1.000000000000000000 ) ) ;
#18149=ORIENTED_EDGE ( 'NONE', *, *, #26487, .F. ) ;
#18153=PLANE ( 'NONE',  #30406 ) ;
#18161=EDGE_CURVE ( 'NONE', #4839, #21061, #28868, .T. ) ;
#18191=VECTOR ( 'NONE', #24760, 1000.000000000000000 ) ;
#18204=CARTESIAN_POINT ( 'NONE',  ( -24.72409385541305582, -14.90920654474426499, 72.98823529411762934 ) ) ;
#18214=DIRECTION ( 'NONE',  ( 3.413470714839332458E-33, -1.190614954331866791E-16, 1.000000000000000000 ) ) ;
#18240=CARTESIAN_POINT ( 'NONE',  ( -50.42609385541305755, -14.80920654474425291, 71.08235294117645253 ) ) ;
#18257=EDGE_CURVE ( 'NONE', #35003, #454, #27358, .T. ) ;
#18259=ORIENTED_EDGE ( 'NONE', *, *, #11815, .F. ) ;
#18276=LINE ( 'NONE', #11157, #19821 ) ;
#18307=ORIENTED_EDGE ( 'NONE', *, *, #9570, .T. ) ;
#18316=ADVANCED_FACE ( 'NONE', ( #37950 ), #31295, .F. ) ;
#18323=EDGE_CURVE ( 'NONE', #41749, #26170, #39164, .T. ) ;
#18335=VERTEX_POINT ( 'NONE', #42643 ) ;
#18357=VERTEX_POINT ( 'NONE', #47298 ) ;
#18389=CARTESIAN_POINT ( 'NONE',  ( -24.72409385541305582, -14.90920654474423124, 69.07058823529411029 ) ) ;
#18421=LINE ( 'NONE', #29771, #4611 ) ;
#18489=ORIENTED_EDGE ( 'NONE', *, *, #13927, .F. ) ;
#18509=LINE ( 'NONE', #35826, #6655 ) ;
#18538=CARTESIAN_POINT ( 'NONE',  ( -24.72409385541305582, -14.90920654474427565, 73.09411764705880898 ) ) ;
#18544=CARTESIAN_POINT ( 'NONE',  ( -24.72409385541305582, -14.80920654474428488, 74.99999999999998579 ) ) ;
#18557=CIRCLE ( 'NONE', #26450, 1.250000000000001110 ) ;
#18591=EDGE_CURVE ( 'NONE', #12927, #27084, #42085, .T. ) ;
#18601=DIRECTION ( 'NONE',  ( 1.000000000000000000, 2.866981220435670867E-17, -3.652049423109068320E-16 ) ) ;
#18606=ORIENTED_EDGE ( 'NONE', *, *, #14082, .F. ) ;
#18610=VERTEX_POINT ( 'NONE', #31962 ) ;
#18616=CARTESIAN_POINT ( 'NONE',  ( -41.18104770156690364, -14.90920654474428630, 72.94436923076921175 ) ) ;
#18618=DIRECTION ( 'NONE',  ( 2.866981220435666553E-17, -1.000000000000000000, -1.190614954331866791E-16 ) ) ;
#18630=VECTOR ( 'NONE', #41430, 1000.000000000000000 ) ;
#18661=VERTEX_POINT ( 'NONE', #46750 ) ;
#18685=ORIENTED_EDGE ( 'NONE', *, *, #24449, .F. ) ;
#18694=VECTOR ( 'NONE', #629, 1000.000000000000000 ) ;
#18743=VERTEX_POINT ( 'NONE', #38870 ) ;
#18774=CARTESIAN_POINT ( 'NONE',  ( -24.72409385541305582, -14.80920654474410902, 57.89999999999999147 ) ) ;
#18805=ORIENTED_EDGE ( 'NONE', *, *, #34007, .F. ) ;
#18821=ADVANCED_FACE ( 'NONE', ( #13942 ), #25784, .T. ) ;
#18839=VECTOR ( 'NONE', #21999, 1000.000000000000000 ) ;
#18884=CARTESIAN_POINT ( 'NONE',  ( -24.72409385541305582, -14.80920654474412679, 59.91176470588234793 ) ) ;
#18918=VECTOR ( 'NONE', #35416, 1000.000000000000000 ) ;
#18937=LINE ( 'NONE', #27298, #38272 ) ;
#18950=VECTOR ( 'NONE', #23120, 1000.000000000000000 ) ;
#18959=FACE_OUTER_BOUND ( 'NONE', #20012, .T. ) ;
#18967=VECTOR ( 'NONE', #27218, 1000.000000000000000 ) ;
#18973=LINE ( 'NONE', #8150, #42472 ) ;
#18977=LINE ( 'NONE', #37925, #25030 ) ;
#18980=FACE_OUTER_BOUND ( 'NONE', #28470, .T. ) ;
#19007=CARTESIAN_POINT ( 'NONE',  ( -50.42409385541305511, -14.80920654474410547, 56.99999999999998579 ) ) ;
#19032=EDGE_CURVE ( 'NONE', #19706, #32553, #35354, .T. ) ;
#19046=CARTESIAN_POINT ( 'NONE',  ( -24.72409385541305582, -14.80920654474412679, 59.91176470588234793 ) ) ;
#19049=FACE_OUTER_BOUND ( 'NONE', #3027, .T. ) ;
#19060=ORIENTED_EDGE ( 'NONE', *, *, #22365, .F. ) ;
#19079=DIRECTION ( 'NONE',  ( -2.866981220435666553E-17, 1.000000000000000000, 1.190614954331866791E-16 ) ) ;
#19120=CARTESIAN_POINT ( 'NONE',  ( -24.72409385541305582, -14.90920654474425255, 71.08235294117645253 ) ) ;
#19125=CYLINDRICAL_SURFACE ( 'NONE', #15464, 1.250000000000001110 ) ;
#19148=CARTESIAN_POINT ( 'NONE',  ( -24.72409385541305582, -14.80920654474421028, 67.05882352941175384 ) ) ;
#19149=EDGE_CURVE ( 'NONE', #27520, #1919, #2823, .T. ) ;
#19150=ADVANCED_FACE ( 'NONE', ( #5815, #32401, #14124 ), #36069, .T. ) ;
#19160=EDGE_CURVE ( 'NONE', #27520, #12228, #24771, .T. ) ;
#19162=DIRECTION ( 'NONE',  ( 1.000000000000000000, 0.000000000000000000, 0.000000000000000000 ) ) ;
#19193=LINE ( 'NONE', #732, #29173 ) ;
#19218=DIRECTION ( 'NONE',  ( -2.866981220435666553E-17, 1.000000000000000000, 1.190614954331866791E-16 ) ) ;
#19219=DIRECTION ( 'NONE',  ( -2.866981220435666553E-17, 1.000000000000000000, 1.190614954331866791E-16 ) ) ;
#19240=ORIENTED_EDGE ( 'NONE', *, *, #1970, .F. ) ;
#19251=CARTESIAN_POINT ( 'NONE',  ( -24.72409385541305582, -14.80920654474410547, 56.99999999999998579 ) ) ;
#19255=DIRECTION ( 'NONE',  ( -2.866981220435666553E-17, 1.000000000000000000, 1.190614954331866791E-16 ) ) ;
#19273=VERTEX_POINT ( 'NONE', #45679 ) ;
#19279=CIRCLE ( 'NONE', #1101, 1.250000000000001110 ) ;
#19286=CARTESIAN_POINT ( 'NONE',  ( -47.17409385541305511, -15.80920654474410725, 70.50000000000000000 ) ) ;
#19299=CARTESIAN_POINT ( 'NONE',  ( -50.42609385541305755, -14.90920654474410512, 56.99999999999998579 ) ) ;
#19334=PLANE ( 'NONE',  #3774 ) ;
#19353=VERTEX_POINT ( 'NONE', #38752 ) ;
#19391=CARTESIAN_POINT ( 'NONE',  ( -41.30484860654427592, -14.90920654474427565, 71.95396199095020506 ) ) ;
#19411=ORIENTED_EDGE ( 'NONE', *, *, #30253, .T. ) ;
#19438=VERTEX_POINT ( 'NONE', #13363 ) ;
#19442=CARTESIAN_POINT ( 'NONE',  ( -24.72409385541305582, -14.80920654474425291, 71.98235294117645822 ) ) ;
#19486=DIRECTION ( 'NONE',  ( -2.866981220435666553E-17, 1.000000000000000000, 1.190614954331866791E-16 ) ) ;
#19495=EDGE_LOOP ( 'NONE', ( #32516, #34149, #18805, #18489, #23148, #14092 ) ) ;
#19496=ADVANCED_FACE ( 'NONE', ( #17052 ), #13599, .T. ) ;
#19504=DIRECTION ( 'NONE',  ( 1.000000000000000000, 2.866981220435666553E-17, 0.000000000000000000 ) ) ;
#19519=LINE ( 'NONE', #8210, #27582 ) ;
#19524=CARTESIAN_POINT ( 'NONE',  ( -50.42609385541305755, -14.80920654474411613, 58.90588235294116970 ) ) ;
#19525=AXIS2_PLACEMENT_3D ( 'NONE', #46316, #20453, #35453 ) ;
#19527=CARTESIAN_POINT ( 'NONE',  ( -24.72409385541305582, -14.80920654474422271, 68.06470588235292496 ) ) ;
#19533=FACE_OUTER_BOUND ( 'NONE', #27738, .T. ) ;
#19559=ORIENTED_EDGE ( 'NONE', *, *, #31239, .F. ) ;
#19573=ADVANCED_FACE ( 'NONE', ( #11380 ), #26403, .T. ) ;
#19602=CARTESIAN_POINT ( 'NONE',  ( -24.72409385541305582, -14.80920654474417830, 64.94117647058821774 ) ) ;
#19653=EDGE_CURVE ( 'NONE', #14295, #37829, #42820, .T. ) ;
#19656=CARTESIAN_POINT ( 'NONE',  ( -46.92409385541305511, -15.80920654474410725, 61.49999999999999289 ) ) ;
#19685=CARTESIAN_POINT ( 'NONE',  ( -41.42864951152165531, -14.90920654474426499, 70.96355475113121258 ) ) ;
#19694=VECTOR ( 'NONE', #7417, 1000.000000000000000 ) ;
#19701=DIRECTION ( 'NONE',  ( 1.000000000000000000, 2.866981220435666553E-17, 0.000000000000000000 ) ) ;
#19706=VERTEX_POINT ( 'NONE', #2169 ) ;
#19747=LINE ( 'NONE', #15784, #10907 ) ;
#19748=VECTOR ( 'NONE', #41179, 1000.000000000000000 ) ;
#19765=VECTOR ( 'NONE', #23151, 1000.000000000000000 ) ;
#19797=ORIENTED_EDGE ( 'NONE', *, *, #26740, .T. ) ;
#19799=EDGE_CURVE ( 'NONE', #41453, #47915, #6600, .T. ) ;
#19801=LINE ( 'NONE', #19299, #46276 ) ;
#19821=VECTOR ( 'NONE', #47615, 1000.000000000000000 ) ;
#19827=ADVANCED_FACE ( 'NONE', ( #40557 ), #17893, .T. ) ;
#19840=LINE ( 'NONE', #12197, #18967 ) ;
#19851=VERTEX_POINT ( 'NONE', #25792 ) ;
#19882=EDGE_CURVE ( 'NONE', #32982, #15059, #25545, .T. ) ;
#19883=VERTEX_POINT ( 'NONE', #18389 ) ;
#19927=DIRECTION ( 'NONE',  ( -3.413470714839332458E-33, 1.190614954331866791E-16, -1.000000000000000000 ) ) ;
#19967=ORIENTED_EDGE ( 'NONE', *, *, #46588, .T. ) ;
#20004=CARTESIAN_POINT ( 'NONE',  ( -41.53953503188365204, -14.90920654474424367, 70.07647058823528141 ) ) ;
#20012=EDGE_LOOP ( 'NONE', ( #229, #3806, #5993, #17627 ) ) ;
#20019=PLANE ( 'NONE',  #47513 ) ;
#20021=DIRECTION ( 'NONE',  ( -2.866981220435666553E-17, 1.000000000000000000, 1.190614954331866791E-16 ) ) ;
#20052=VECTOR ( 'NONE', #10476, 1000.000000000000000 ) ;
#20053=ADVANCED_FACE ( 'NONE', ( #19533 ), #34295, .T. ) ;
#20067=DIRECTION ( 'NONE',  ( 2.866981220435666553E-17, -1.000000000000000000, -1.190614954331866791E-16 ) ) ;
#20073=CARTESIAN_POINT ( 'NONE',  ( -24.72409385541305582, -14.90920654474412643, 59.01176470588234224 ) ) ;
#20155=LINE ( 'NONE', #8850, #35745 ) ;
#20207=CARTESIAN_POINT ( 'NONE',  ( -24.72409385541305582, -15.80920654474410725, 65.99999999999998579 ) ) ;
#20209=LINE ( 'NONE', #1245, #28169 ) ;
#20221=VECTOR ( 'NONE', #33147, 1000.000000000000000 ) ;
#20223=VECTOR ( 'NONE', #28152, 1000.000000000000000 ) ;
#20227=VECTOR ( 'NONE', #42952, 1000.000000000000114 ) ;
#20250=LINE ( 'NONE', #8044, #25772 ) ;
#20287=LINE ( 'NONE', #8732, #20611 ) ;
#20299=LINE ( 'NONE', #16588, #2509 ) ;
#20305=LINE ( 'NONE', #27928, #20227 ) ;
#20310=CARTESIAN_POINT ( 'NONE',  ( -42.67115267894247665, -14.80920654474414810, 61.02352941176469869 ) ) ;
#20342=ORIENTED_EDGE ( 'NONE', *, *, #39122, .T. ) ;
#20368=CARTESIAN_POINT ( 'NONE',  ( -41.92997620835424044, -14.80920654474420139, 66.95294117647057419 ) ) ;
#20397=PLANE ( 'NONE',  #47913 ) ;
#20403=AXIS2_PLACEMENT_3D ( 'NONE', #6221, #28397, #43422 ) ;
#20411=VECTOR ( 'NONE', #15041, 1000.000000000000114 ) ;
#20423=ORIENTED_EDGE ( 'NONE', *, *, #45828, .T. ) ;
#20425=CARTESIAN_POINT ( 'NONE',  ( -24.72409385541305582, -15.80920654474410725, 65.99999999999998579 ) ) ;
#20453=DIRECTION ( 'NONE',  ( -0.9922778767136676281, -4.321618136576820974E-17, 0.1240347345892086200 ) ) ;
#20457=AXIS2_PLACEMENT_3D ( 'NONE', #950, #34672, #15212 ) ;
#20465=FACE_OUTER_BOUND ( 'NONE', #40885, .T. ) ;
#20475=VECTOR ( 'NONE', #21873, 1000.000000000000000 ) ;
#20484=CARTESIAN_POINT ( 'NONE',  ( -41.67850562011894766, -14.90920654474422058, 68.96470588235293064 ) ) ;
#20546=VECTOR ( 'NONE', #1381, 1000.000000000000000 ) ;
#20555=EDGE_CURVE ( 'NONE', #45977, #7144, #12009, .T. ) ;
#20591=ADVANCED_FACE ( 'NONE', ( #27504 ), #40509, .T. ) ;
#20611=VECTOR ( 'NONE', #23760, 1000.000000000000000 ) ;
#20634=ORIENTED_EDGE ( 'NONE', *, *, #34639, .F. ) ;
#20638=ORIENTED_EDGE ( 'NONE', *, *, #38111, .F. ) ;
#20640=FACE_OUTER_BOUND ( 'NONE', #24104, .T. ) ;
#20641=ORIENTED_EDGE ( 'NONE', *, *, #25759, .T. ) ;
#20697=VECTOR ( 'NONE', #25458, 1000.000000000000000 ) ;
#20728=CARTESIAN_POINT ( 'NONE',  ( -24.72409385541305582, -14.80920654474421205, 67.95882352941174531 ) ) ;
#20744=ORIENTED_EDGE ( 'NONE', *, *, #5878, .F. ) ;
#20762=CARTESIAN_POINT ( 'NONE',  ( -50.42609385541305755, -14.80920654474426534, 72.08823529411763786 ) ) ;
#20803=VERTEX_POINT ( 'NONE', #26725 ) ;
#20804=CARTESIAN_POINT ( 'NONE',  ( -50.42609385541305755, -14.90920654474423301, 69.07058823529411029 ) ) ;
#20826=DIRECTION ( 'NONE',  ( -0.1240347345892086062, 1.145860353393066553E-16, -0.9922778767136676281 ) ) ;
#20839=ORIENTED_EDGE ( 'NONE', *, *, #16695, .F. ) ;
#20847=DIRECTION ( 'NONE',  ( 1.000000000000000000, 2.866981220435666553E-17, 0.000000000000000000 ) ) ;
#20889=ORIENTED_EDGE ( 'NONE', *, *, #32580, .F. ) ;
#20922=ORIENTED_EDGE ( 'NONE', *, *, #18323, .F. ) ;
#20965=ORIENTED_EDGE ( 'NONE', *, *, #28339, .T. ) ;
#20984=LINE ( 'NONE', #13572, #21542 ) ;
#21022=DIRECTION ( 'NONE',  ( 1.000000000000000000, 2.866981220435666553E-17, 0.000000000000000000 ) ) ;
#21024=CARTESIAN_POINT ( 'NONE',  ( -50.42409385541305511, -14.80920654474410725, 74.99999999999998579 ) ) ;
#21028=VERTEX_POINT ( 'NONE', #40694 ) ;
#21055=CARTESIAN_POINT ( 'NONE',  ( -41.80005222645378637, -14.90920654474423124, 67.99233303167419251 ) ) ;
#21059=ORIENTED_EDGE ( 'NONE', *, *, #5790, .F. ) ;
#21061=VERTEX_POINT ( 'NONE', #41427 ) ;
#21132=DIRECTION ( 'NONE',  ( -2.866981220435666553E-17, 1.000000000000000000, 1.190614954331866791E-16 ) ) ;
#21145=AXIS2_PLACEMENT_3D ( 'NONE', #3208, #18214, #14738 ) ;
#21155=DIRECTION ( 'NONE',  ( 2.866981220435666553E-17, -1.000000000000000000, -1.190614954331866791E-16 ) ) ;
#21165=ORIENTED_EDGE ( 'NONE', *, *, #23609, .F. ) ;
#21168=VECTOR ( 'NONE', #13249, 1000.000000000000000 ) ;
#21235=DIRECTION ( 'NONE',  ( -2.866981220435666553E-17, 1.000000000000000000, 1.190614954331866791E-16 ) ) ;
#21239=EDGE_LOOP ( 'NONE', ( #25619, #35829 ) ) ;
#21259=FACE_OUTER_BOUND ( 'NONE', #16453, .T. ) ;
#21270=LINE ( 'NONE', #2553, #22514 ) ;
#21276=PLANE ( 'NONE',  #22273 ) ;
#21278=VECTOR ( 'NONE', #37178, 1000.000000000000000 ) ;
#21303=EDGE_CURVE ( 'NONE', #42385, #21562, #6908, .T. ) ;
#21305=CYLINDRICAL_SURFACE ( 'NONE', #9409, 1.250000000000001110 ) ;
#21314=CARTESIAN_POINT ( 'NONE',  ( -40.92409385541305511, -15.80920654474410725, 74.99999999999998579 ) ) ;
#21346=ORIENTED_EDGE ( 'NONE', *, *, #20555, .T. ) ;
#21352=LINE ( 'NONE', #47448, #39332 ) ;
#21415=VERTEX_POINT ( 'NONE', #9285 ) ;
#21423=CARTESIAN_POINT ( 'NONE',  ( -24.72409385541305582, -14.80920654474418896, 65.04705882352939739 ) ) ;
#21427=PLANE ( 'NONE',  #7010 ) ;
#21431=ORIENTED_EDGE ( 'NONE', *, *, #30733, .F. ) ;
#21469=VECTOR ( 'NONE', #44905, 1000.000000000000114 ) ;
#21499=DIRECTION ( 'NONE',  ( 2.866981220435666553E-17, -1.000000000000000000, -1.190614954331866791E-16 ) ) ;
#21508=DIRECTION ( 'NONE',  ( 3.413470714839332458E-33, -1.190614954331866791E-16, 1.000000000000000000 ) ) ;
#21520=LINE ( 'NONE', #14087, #21469 ) ;
#21534=DIRECTION ( 'NONE',  ( 2.866981220435666553E-17, -1.000000000000000000, -1.190614954331866791E-16 ) ) ;
#21542=VECTOR ( 'NONE', #35267, 1000.000000000000000 ) ;
#21562=VERTEX_POINT ( 'NONE', #21807 ) ;
#21641=DIRECTION ( 'NONE',  ( 1.000000000000000000, 2.866981220435666553E-17, 0.000000000000000000 ) ) ;
#21644=LINE ( 'NONE', #45285, #7768 ) ;
#21648=EDGE_CURVE ( 'NONE', #24654, #5607, #15369, .T. ) ;
#21766=ORIENTED_EDGE ( 'NONE', *, *, #31095, .F. ) ;
#21784=CARTESIAN_POINT ( 'NONE',  ( -40.92409385541305511, -14.80920654474410725, 74.99999999999998579 ) ) ;
#21807=CARTESIAN_POINT ( 'NONE',  ( -24.72409385541305582, -14.90920654474414775, 61.92352941176469727 ) ) ;
#21826=DIRECTION ( 'NONE',  ( 1.000000000000000000, 0.000000000000000000, 0.000000000000000000 ) ) ;
#21830=ORIENTED_EDGE ( 'NONE', *, *, #40567, .T. ) ;
#21843=LINE ( 'NONE', #18132, #20221 ) ;
#21873=DIRECTION ( 'NONE',  ( 3.413470714839332458E-33, -1.190614954331866791E-16, 1.000000000000000000 ) ) ;
#21903=AXIS2_PLACEMENT_3D ( 'NONE', #8720, #38740, #8234 ) ;
#21910=CARTESIAN_POINT ( 'NONE',  ( -24.72409385541305582, -14.90920654474416729, 63.03529411764704804 ) ) ;
#21913=VERTEX_POINT ( 'NONE', #40242 ) ;
#21935=ORIENTED_EDGE ( 'NONE', *, *, #18257, .F. ) ;
#21982=ORIENTED_EDGE ( 'NONE', *, *, #17838, .T. ) ;
#21993=VECTOR ( 'NONE', #22144, 1000.000000000000114 ) ;
#21999=DIRECTION ( 'NONE',  ( 2.866981220435666553E-17, -1.000000000000000000, -1.190614954331866791E-16 ) ) ;
#22028=LINE ( 'NONE', #21314, #41211 ) ;
#22034=CARTESIAN_POINT ( 'NONE',  ( -50.42609385541305755, -14.90920654474412643, 59.91176470588234793 ) ) ;
#22041=ORIENTED_EDGE ( 'NONE', *, *, #10495, .T. ) ;
#22054=ORIENTED_EDGE ( 'NONE', *, *, #1561, .T. ) ;
#22065=CARTESIAN_POINT ( 'NONE',  ( -42.79688797306012304, -14.90920654474413709, 60.01764705882352047 ) ) ;
#22074=ORIENTED_EDGE ( 'NONE', *, *, #2957, .T. ) ;
#22075=DIRECTION ( 'NONE',  ( 2.866981220435666553E-17, -1.000000000000000000, -1.190614954331866791E-16 ) ) ;
#22078=VECTOR ( 'NONE', #47744, 1000.000000000000000 ) ;
#22107=( GEOMETRIC_REPRESENTATION_CONTEXT ( 3 ) GLOBAL_UNCERTAINTY_ASSIGNED_CONTEXT ( ( #13460 ) ) GLOBAL_UNIT_ASSIGNED_CONTEXT ( ( #5412, #33349, #47260 ) ) REPRESENTATION_CONTEXT ( 'NONE', 'WORKASPACE' ) );
#22108=CARTESIAN_POINT ( 'NONE',  ( -24.72409385541305582, -14.80920654474413745, 60.91764705882351905 ) ) ;
#22129=VECTOR ( 'NONE', #33781, 1000.000000000000000 ) ;
#22137=ORIENTED_EDGE ( 'NONE', *, *, #23870, .T. ) ;
#22144=DIRECTION ( 'NONE',  ( -0.1240347345892086062, 1.145860353393066553E-16, -0.9922778767136676281 ) ) ;
#22191=CARTESIAN_POINT ( 'NONE',  ( -50.42609385541305755, -14.80920654474412679, 59.01176470588234224 ) ) ;
#22236=CARTESIAN_POINT ( 'NONE',  ( -24.72409385541305582, -14.80920654474413745, 60.91764705882351905 ) ) ;
#22240=EDGE_LOOP ( 'NONE', ( #15749, #41532, #16639, #13571 ) ) ;
#22253=ORIENTED_EDGE ( 'NONE', *, *, #26053, .F. ) ;
#22273=AXIS2_PLACEMENT_3D ( 'NONE', #21024, #1579, #43690 ) ;
#22285=EDGE_CURVE ( 'NONE', #46722, #12016, #13081, .T. ) ;
#22311=ORIENTED_EDGE ( 'NONE', *, *, #1916, .F. ) ;
#22339=VECTOR ( 'NONE', #29288, 1000.000000000000000 ) ;
#22365=EDGE_CURVE ( 'NONE', #1410, #47208, #31515, .T. ) ;
#22384=EDGE_LOOP ( 'NONE', ( #4322, #47150, #24531, #41254 ) ) ;
#22387=CARTESIAN_POINT ( 'NONE',  ( -50.42609385541305755, -14.80920654474418008, 64.04117647058822627 ) ) ;
#22406=DIRECTION ( 'NONE',  ( 1.000000000000000000, 0.000000000000000000, 0.000000000000000000 ) ) ;
#22419=DIRECTION ( 'NONE',  ( -2.866981220435666553E-17, 1.000000000000000000, 1.190614954331866791E-16 ) ) ;
#22438=ADVANCED_FACE ( 'NONE', ( #45820 ), #509, .T. ) ;
#22466=DIRECTION ( 'NONE',  ( -2.866981220435666553E-17, 1.000000000000000000, 1.190614954331866791E-16 ) ) ;
#22472=EDGE_CURVE ( 'NONE', #5607, #19438, #18557, .T. ) ;
#22495=VERTEX_POINT ( 'NONE', #15750 ) ;
#22514=VECTOR ( 'NONE', #21022, 1000.000000000000000 ) ;
#22576=CARTESIAN_POINT ( 'NONE',  ( -45.92409385541305511, -15.81020654474410847, 70.50000000000000000 ) ) ;
#22618=VERTEX_POINT ( 'NONE', #44541 ) ;
#22646=DIRECTION ( 'NONE',  ( -0.1240347345892086200, 1.145860353393066553E-16, -0.9922778767136676281 ) ) ;
#22665=VERTEX_POINT ( 'NONE', #36629 ) ;
#22689=VECTOR ( 'NONE', #25473, 1000.000000000000114 ) ;
#22728=EDGE_CURVE ( 'NONE', #20803, #22914, #27036, .T. ) ;
#22779=AXIS2_PLACEMENT_3D ( 'NONE', #40009, #46912, #44213 ) ;
#22788=EDGE_CURVE ( 'NONE', #2135, #18357, #42202, .T. ) ;
#22808=ORIENTED_EDGE ( 'NONE', *, *, #28736, .T. ) ;
#22838=VECTOR ( 'NONE', #23165, 1000.000000000000000 ) ;
#22848=ORIENTED_EDGE ( 'NONE', *, *, #12988, .F. ) ;
#22858=EDGE_LOOP ( 'NONE', ( #9232, #21766, #12970, #8471, #41805, #12092 ) ) ;
#22861=ADVANCED_FACE ( 'NONE', ( #2137 ), #36102, .T. ) ;
#22879=PRODUCT_DEFINITION_SHAPE ( 'NONE', 'NONE',  #42442 ) ;
#22880=DIRECTION ( 'NONE',  ( 2.866981220435666553E-17, -1.000000000000000000, -1.190614954331866791E-16 ) ) ;
#22893=ORIENTED_EDGE ( 'NONE', *, *, #38809, .T. ) ;
#22907=VECTOR ( 'NONE', #12234, 1000.000000000000000 ) ;
#22914=VERTEX_POINT ( 'NONE', #19046 ) ;
#22931=DIRECTION ( 'NONE',  ( -3.413470714839332458E-33, 1.190614954331866791E-16, -1.000000000000000000 ) ) ;
#22947=LINE ( 'NONE', #45832, #1917 ) ;
#22948=CARTESIAN_POINT ( 'NONE',  ( -24.72409385541305582, -14.80920654474426357, 72.98823529411762934 ) ) ;
#22968=DIRECTION ( 'NONE',  ( -0.1240347345892086062, 1.145860353393066553E-16, -0.9922778767136676281 ) ) ;
#23016=VERTEX_POINT ( 'NONE', #19442 ) ;
#23042=DIRECTION ( 'NONE',  ( 1.000000000000000000, 2.866981220435666553E-17, 0.000000000000000000 ) ) ;
#23107=DIRECTION ( 'NONE',  ( -2.866981220435666553E-17, 1.000000000000000000, 1.190614954331866791E-16 ) ) ;
#23113=DIRECTION ( 'NONE',  ( 3.413470714839332458E-33, -1.190614954331866791E-16, 1.000000000000000000 ) ) ;
#23120=DIRECTION ( 'NONE',  ( 1.000000000000000000, 2.866981220435666553E-17, 0.000000000000000000 ) ) ;
#23129=ORIENTED_EDGE ( 'NONE', *, *, #43485, .T. ) ;
#23145=( NAMED_UNIT ( * ) SI_UNIT ( $, .STERADIAN. ) SOLID_ANGLE_UNIT ( ) );
#23148=ORIENTED_EDGE ( 'NONE', *, *, #47238, .F. ) ;
#23151=DIRECTION ( 'NONE',  ( -2.866981220435666553E-17, 1.000000000000000000, 1.190614954331866791E-16 ) ) ;
#23165=DIRECTION ( 'NONE',  ( -3.413470714839332458E-33, 1.190614954331866791E-16, -1.000000000000000000 ) ) ;
#23168=CARTESIAN_POINT ( 'NONE',  ( -43.17409385541305511, -14.80920654474410547, 56.99999999999998579 ) ) ;
#23170=DIRECTION ( 'NONE',  ( -2.866981220435666553E-17, 1.000000000000000000, 1.190614954331866791E-16 ) ) ;
#23177=DIRECTION ( 'NONE',  ( 2.866981220435666553E-17, -1.000000000000000000, -1.190614954331866791E-16 ) ) ;
#23205=DIRECTION ( 'NONE',  ( -3.413470714839332458E-33, 1.190614954331866791E-16, -1.000000000000000000 ) ) ;
#23229=CARTESIAN_POINT ( 'NONE',  ( -24.72409385541305582, -14.90920654474417972, 64.94117647058821774 ) ) ;
#23231=FACE_OUTER_BOUND ( 'NONE', #12247, .T. ) ;
#23233=LINE ( 'NONE', #18538, #12392 ) ;
#23236=DIRECTION ( 'NONE',  ( 1.000000000000000000, 2.866981220435666553E-17, 0.000000000000000000 ) ) ;
#23249=CARTESIAN_POINT ( 'NONE',  ( -50.42609385541305755, -14.80920654474422271, 68.96470588235293064 ) ) ;
#23274=PLANE ( 'NONE',  #41819 ) ;
#23275=EDGE_CURVE ( 'NONE', #23280, #41320, #26064, .T. ) ;
#23280=VERTEX_POINT ( 'NONE', #19148 ) ;
#23289=ORIENTED_EDGE ( 'NONE', *, *, #954, .F. ) ;
#23301=DIRECTION ( 'NONE',  ( -2.866981220435666553E-17, 1.000000000000000000, 1.190614954331866791E-16 ) ) ;
#23375=CARTESIAN_POINT ( 'NONE',  ( -24.72409385541305582, -14.90920654474424190, 70.07647058823528141 ) ) ;
#23383=LINE ( 'NONE', #41860, #19765 ) ;
#23406=PLANE ( 'NONE',  #2973 ) ;
#23427=VECTOR ( 'NONE', #32420, 1000.000000000000000 ) ;
#23434=CARTESIAN_POINT ( 'NONE',  ( -50.42609385541305755, -14.80920654474420139, 66.05294117647058272 ) ) ;
#23454=LINE ( 'NONE', #12359, #9372 ) ;
#23489=ORIENTED_EDGE ( 'NONE', *, *, #37483, .T. ) ;
#23509=VERTEX_POINT ( 'NONE', #20368 ) ;
#23512=CARTESIAN_POINT ( 'NONE',  ( -50.42609385541305755, -14.90920654474410512, 57.89999999999999147 ) ) ;
#23520=CARTESIAN_POINT ( 'NONE',  ( -24.72409385541305582, -15.80920654474410725, 65.99999999999998579 ) ) ;
#23526=EDGE_CURVE ( 'NONE', #25093, #11434, #47440, .T. ) ;
#23547=ORIENTED_EDGE ( 'NONE', *, *, #25292, .F. ) ;
#23597=CARTESIAN_POINT ( 'NONE',  ( -24.72409385541305582, -14.80920654474412679, 59.91176470588234793 ) ) ;
#23603=ORIENTED_EDGE ( 'NONE', *, *, #6200, .T. ) ;
#23607=DIRECTION ( 'NONE',  ( 1.000000000000000000, 2.866981220435666553E-17, 0.000000000000000000 ) ) ;
#23609=EDGE_CURVE ( 'NONE', #48232, #47529, #40759, .T. ) ;
#23638=ORIENTED_EDGE ( 'NONE', *, *, #21648, .F. ) ;
#23738=VECTOR ( 'NONE', #39693, 1000.000000000000000 ) ;
#23760=DIRECTION ( 'NONE',  ( -2.866981220435666553E-17, 1.000000000000000000, 1.190614954331866791E-16 ) ) ;
#23772=CARTESIAN_POINT ( 'NONE',  ( -24.72409385541305582, -14.80920654474413745, 60.01764705882352047 ) ) ;
#23807=EDGE_CURVE ( 'NONE', #19706, #40467, #45930, .T. ) ;
#23847=EDGE_LOOP ( 'NONE', ( #8531, #36471, #38259, #10702 ) ) ;
#23864=LINE ( 'NONE', #5144, #38497 ) ;
#23870=EDGE_CURVE ( 'NONE', #18335, #24420, #24256, .T. ) ;
#23901=VECTOR ( 'NONE', #757, 1000.000000000000000 ) ;
#23914=EDGE_LOOP ( 'NONE', ( #2731, #9510 ) ) ;
#23915=ORIENTED_EDGE ( 'NONE', *, *, #25222, .F. ) ;
#23929=CARTESIAN_POINT ( 'NONE',  ( -24.72409385541305582, -14.80920654474423159, 69.97058823529410176 ) ) ;
#23934=ORIENTED_EDGE ( 'NONE', *, *, #44575, .T. ) ;
#23944=EDGE_CURVE ( 'NONE', #10723, #31686, #25456, .T. ) ;
#23957=CARTESIAN_POINT ( 'NONE',  ( -46.92409385541305511, -15.81020654474410847, 61.49999999999999289 ) ) ;
#23960=LINE ( 'NONE', #45396, #47854 ) ;
#23962=CARTESIAN_POINT ( 'NONE',  ( -50.42609385541305755, -14.80920654474410902, 57.89999999999999147 ) ) ;
#24003=DIRECTION ( 'NONE',  ( 1.000000000000000000, 2.866981220435666553E-17, 0.000000000000000000 ) ) ;
#24038=VERTEX_POINT ( 'NONE', #41692 ) ;
#24104=EDGE_LOOP ( 'NONE', ( #39761, #33295, #27827, #31673 ) ) ;
#24120=CARTESIAN_POINT ( 'NONE',  ( -24.72409385541305582, -14.90920654474412643, 59.91176470588234793 ) ) ;
#24126=VERTEX_POINT ( 'NONE', #23229 ) ;
#24136=LINE ( 'NONE', #9362, #14727 ) ;
#24150=ORIENTED_EDGE ( 'NONE', *, *, #1970, .T. ) ;
#24230=VERTEX_POINT ( 'NONE', #16290 ) ;
#24237=VERTEX_POINT ( 'NONE', #9175 ) ;
#24245=VECTOR ( 'NONE', #38340, 1000.000000000000114 ) ;
#24256=LINE ( 'NONE', #20310, #9291 ) ;
#24348=ORIENTED_EDGE ( 'NONE', *, *, #13669, .F. ) ;
#24371=VECTOR ( 'NONE', #36147, 1000.000000000000114 ) ;
#24377=VECTOR ( 'NONE', #12710, 1000.000000000000000 ) ;
#24387=ADVANCED_FACE ( 'NONE', ( #45097 ), #23406, .F. ) ;
#24405=DIRECTION ( 'NONE',  ( -3.413470714839332458E-33, 1.190614954331866791E-16, -1.000000000000000000 ) ) ;
#24420=VERTEX_POINT ( 'NONE', #27091 ) ;
#24423=PLANE ( 'NONE',  #2476 ) ;
#24425=VECTOR ( 'NONE', #41474, 1000.000000000000114 ) ;
#24430=CARTESIAN_POINT ( 'NONE',  ( -41.28806444364835215, -14.90920654474426499, 72.08823529411763786 ) ) ;
#24449=EDGE_CURVE ( 'NONE', #21913, #43447, #18977, .T. ) ;
#24454=AXIS2_PLACEMENT_3D ( 'NONE', #13665, #28712, #35840 ) ;
#24463=CARTESIAN_POINT ( 'NONE',  ( -50.42609385541305755, -14.90920654474423301, 69.07058823529411029 ) ) ;
#24477=FACE_OUTER_BOUND ( 'NONE', #42635, .T. ) ;
#24531=ORIENTED_EDGE ( 'NONE', *, *, #13142, .T. ) ;
#24563=ORIENTED_EDGE ( 'NONE', *, *, #26736, .T. ) ;
#24583=ORIENTED_EDGE ( 'NONE', *, *, #31158, .F. ) ;
#24613=DIRECTION ( 'NONE',  ( 3.413470714839332458E-33, -1.190614954331866791E-16, 1.000000000000000000 ) ) ;
#24652=CARTESIAN_POINT ( 'NONE',  ( -41.92385313143115155, -14.90920654474422058, 67.00192579185520003 ) ) ;
#24654=VERTEX_POINT ( 'NONE', #14394 ) ;
#24683=CARTESIAN_POINT ( 'NONE',  ( -45.92409385541305511, -15.81020654474410847, 70.50000000000000000 ) ) ;
#24690=DIRECTION ( 'NONE',  ( 3.413470714839332458E-33, -1.190614954331866791E-16, 1.000000000000000000 ) ) ;
#24705=FACE_OUTER_BOUND ( 'NONE', #27488, .T. ) ;
#24722=DIRECTION ( 'NONE',  ( -0.1240347345892086062, 1.145860353393066553E-16, -0.9922778767136676281 ) ) ;
#24735=DIRECTION ( 'NONE',  ( -6.867234345585435779E-33, 2.395284034871316381E-16, -1.000000000000000000 ) ) ;
#24760=DIRECTION ( 'NONE',  ( 2.866981220435666553E-17, -1.000000000000000000, -1.190614954331866791E-16 ) ) ;
#24771=LINE ( 'NONE', #21784, #41667 ) ;
#24782=CARTESIAN_POINT ( 'NONE',  ( -50.42609385541305755, -14.80920654474424225, 70.97647058823527288 ) ) ;
#24799=VERTEX_POINT ( 'NONE', #8049 ) ;
#24858=ORIENTED_EDGE ( 'NONE', *, *, #47661, .F. ) ;
#24878=LINE ( 'NONE', #39892, #6923 ) ;
#24917=DIRECTION ( 'NONE',  ( 1.000000000000000000, 2.866981220435670867E-17, -3.652049423109068320E-16 ) ) ;
#24925=CARTESIAN_POINT ( 'NONE',  ( -24.72409385541305582, -15.80920654474410725, 65.99999999999998579 ) ) ;
#24928=ORIENTED_EDGE ( 'NONE', *, *, #17911, .F. ) ;
#24934=CARTESIAN_POINT ( 'NONE',  ( -24.72409385541305582, -15.80920654474410725, 65.99999999999998579 ) ) ;
#24942=AXIS2_PLACEMENT_3D ( 'NONE', #16745, #38688, #8664 ) ;
#24991=ORIENTED_EDGE ( 'NONE', *, *, #23609, .T. ) ;
#25000=ORIENTED_EDGE ( 'NONE', *, *, #41438, .F. ) ;
#25003=VECTOR ( 'NONE', #35069, 1000.000000000000000 ) ;
#25012=EDGE_CURVE ( 'NONE', #46722, #37730, #40717, .T. ) ;
#25014=VECTOR ( 'NONE', #41391, 1000.000000000000000 ) ;
#25030=VECTOR ( 'NONE', #12078, 1000.000000000000114 ) ;
#25041=ADVANCED_FACE ( 'NONE', ( #29897 ), #48111, .T. ) ;
#25088=ORIENTED_EDGE ( 'NONE', *, *, #11527, .F. ) ;
#25090=PLANE ( 'NONE',  #38448 ) ;
#25093=VERTEX_POINT ( 'NONE', #42436 ) ;
#25105=VERTEX_POINT ( 'NONE', #19286 ) ;
#25113=CARTESIAN_POINT ( 'NONE',  ( -24.72409385541305582, -15.80920654474410725, 65.99999999999998579 ) ) ;
#25133=DIRECTION ( 'NONE',  ( 2.866981220435666553E-17, -1.000000000000000000, -1.190614954331866791E-16 ) ) ;
#25147=AXIS2_PLACEMENT_3D ( 'NONE', #2286, #32343, #47365 ) ;
#25184=PLANE ( 'NONE',  #45472 ) ;
#25212=ORIENTED_EDGE ( 'NONE', *, *, #26564, .F. ) ;
#25220=VERTEX_POINT ( 'NONE', #45400 ) ;
#25222=EDGE_CURVE ( 'NONE', #32553, #23280, #41944, .T. ) ;
#25223=LINE ( 'NONE', #40248, #2951 ) ;
#25229=DIRECTION ( 'NONE',  ( 2.866981220435666553E-17, -1.000000000000000000, -1.190614954331866791E-16 ) ) ;
#25233=VECTOR ( 'NONE', #45388, 1000.000000000000000 ) ;
#25236=FACE_OUTER_BOUND ( 'NONE', #8828, .T. ) ;
#25242=DIRECTION ( 'NONE',  ( -2.866981220435666553E-17, 1.000000000000000000, 1.190614954331866791E-16 ) ) ;
#25292=EDGE_CURVE ( 'NONE', #17265, #18661, #2265, .T. ) ;
#25307=LINE ( 'NONE', #18616, #47825 ) ;
#25317=VECTOR ( 'NONE', #21132, 1000.000000000000000 ) ;
#25323=ORIENTED_EDGE ( 'NONE', *, *, #48078, .F. ) ;
#25353=CARTESIAN_POINT ( 'NONE',  ( -50.42609385541305755, -14.80920654474428666, 74.09999999999998010 ) ) ;
#25390=EDGE_LOOP ( 'NONE', ( #2904, #11569, #5949, #1680 ) ) ;
#25408=DIRECTION ( 'NONE',  ( -3.413470714839332458E-33, 1.190614954331866791E-16, -1.000000000000000000 ) ) ;
#25428=EDGE_LOOP ( 'NONE', ( #41354, #44181, #37961, #28717 ) ) ;
#25438=ORIENTED_EDGE ( 'NONE', *, *, #22472, .T. ) ;
#25456=LINE ( 'NONE', #40958, #2179 ) ;
#25458=DIRECTION ( 'NONE',  ( -2.866981220435666553E-17, 1.000000000000000000, 1.190614954331866791E-16 ) ) ;
#25473=DIRECTION ( 'NONE',  ( -0.1240347345892086200, 1.145860353393066553E-16, -0.9922778767136676281 ) ) ;
#25491=ADVANCED_FACE ( 'NONE', ( #17745 ), #44143, .T. ) ;
#25520=LINE ( 'NONE', #29461, #12421 ) ;
#25524=CARTESIAN_POINT ( 'NONE',  ( -42.91426037125016535, -14.90920654474413709, 59.07866787330315361 ) ) ;
#25545=LINE ( 'NONE', #22108, #3161 ) ;
#25563=DIRECTION ( 'NONE',  ( 2.866981220435666553E-17, -1.000000000000000000, -1.190614954331866791E-16 ) ) ;
#25587=ORIENTED_EDGE ( 'NONE', *, *, #23526, .F. ) ;
#25609=EDGE_CURVE ( 'NONE', #16499, #40821, #38409, .T. ) ;
#25612=EDGE_CURVE ( 'NONE', #46946, #23016, #7925, .T. ) ;
#25619=ORIENTED_EDGE ( 'NONE', *, *, #22472, .F. ) ;
#25620=LINE ( 'NONE', #13558, #7109 ) ;
#25651=DIRECTION ( 'NONE',  ( 2.866981220435666553E-17, -1.000000000000000000, -1.190614954331866791E-16 ) ) ;
#25659=DIRECTION ( 'NONE',  ( -0.1240347345892086062, 1.145860353393066553E-16, -0.9922778767136676281 ) ) ;
#25699=VECTOR ( 'NONE', #13307, 1000.000000000000000 ) ;
#25716=ORIENTED_EDGE ( 'NONE', *, *, #36464, .T. ) ;
#25717=ORIENTED_EDGE ( 'NONE', *, *, #39122, .F. ) ;
#25727=EDGE_CURVE ( 'NONE', #15919, #15234, #18421, .T. ) ;
#25738=CARTESIAN_POINT ( 'NONE',  ( -50.42609385541305755, -14.90920654474411577, 58.90588235294116970 ) ) ;
#25751=ORIENTED_EDGE ( 'NONE', *, *, #32580, .T. ) ;
#25759=EDGE_CURVE ( 'NONE', #24420, #46610, #32948, .T. ) ;
#25772=VECTOR ( 'NONE', #17014, 1000.000000000000000 ) ;
#25781=VECTOR ( 'NONE', #36456, 1000.000000000000000 ) ;
#25784=PLANE ( 'NONE',  #47183 ) ;
#25788=EDGE_LOOP ( 'NONE', ( #10776, #22137, #14646, #45805 ) ) ;
#25792=CARTESIAN_POINT ( 'NONE',  ( -43.04835856129541583, -14.90920654474411577, 58.00588235294116402 ) ) ;
#25796=ORIENTED_EDGE ( 'NONE', *, *, #10220, .T. ) ;
#25892=ORIENTED_EDGE ( 'NONE', *, *, #7660, .F. ) ;
#25915=DIRECTION ( 'NONE',  ( 1.000000000000000000, 2.866981220435666553E-17, 0.000000000000000000 ) ) ;
#25951=EDGE_CURVE ( 'NONE', #7670, #38928, #9561, .T. ) ;
#25953=CARTESIAN_POINT ( 'NONE',  ( -24.72409385541305582, -14.90920654474422058, 68.06470588235292496 ) ) ;
#25993=AXIS2_PLACEMENT_3D ( 'NONE', #27914, #42937, #5522 ) ;
#26022=ORIENTED_EDGE ( 'NONE', *, *, #34637, .F. ) ;
#26053=EDGE_CURVE ( 'NONE', #31211, #12927, #47694, .T. ) ;
#26054=FACE_OUTER_BOUND ( 'NONE', #6226, .T. ) ;
#26064=LINE ( 'NONE', #26297, #10721 ) ;
#26078=ORIENTED_EDGE ( 'NONE', *, *, #13669, .T. ) ;
#26081=DIRECTION ( 'NONE',  ( -3.413470714839332458E-33, 1.190614954331866791E-16, -1.000000000000000000 ) ) ;
#26083=ORIENTED_EDGE ( 'NONE', *, *, #11527, .T. ) ;
#26127=ORIENTED_EDGE ( 'NONE', *, *, #2032, .T. ) ;
#26148=ORIENTED_EDGE ( 'NONE', *, *, #954, .T. ) ;
#26169=FACE_OUTER_BOUND ( 'NONE', #27207, .T. ) ;
#26170=VERTEX_POINT ( 'NONE', #48664 ) ;
#26211=LINE ( 'NONE', #45423, #41678 ) ;
#26228=ADVANCED_FACE ( 'NONE', ( #37563 ), #30219, .T. ) ;
#26297=CARTESIAN_POINT ( 'NONE',  ( -24.72409385541305582, -14.80920654474421205, 67.95882352941174531 ) ) ;
#26327=DIRECTION ( 'NONE',  ( 2.866981220435666553E-17, -1.000000000000000000, -1.190614954331866791E-16 ) ) ;
#26363=LINE ( 'NONE', #45591, #27791 ) ;
#26372=CARTESIAN_POINT ( 'NONE',  ( -24.72409385541305582, -14.90920654474420104, 66.95294117647057419 ) ) ;
#26374=LINE ( 'NONE', #11599, #25014 ) ;
#26379=ORIENTED_EDGE ( 'NONE', *, *, #33522, .T. ) ;
#26403=PLANE ( 'NONE',  #3996 ) ;
#26445=LINE ( 'NONE', #30156, #46526 ) ;
#26450=AXIS2_PLACEMENT_3D ( 'NONE', #4209, #19218, #34220 ) ;
#26453=DIRECTION ( 'NONE',  ( 1.000000000000000000, 2.866981220435666553E-17, 0.000000000000000000 ) ) ;
#26462=CARTESIAN_POINT ( 'NONE',  ( -43.03806127622754474, -14.90920654474412643, 58.08826063348414692 ) ) ;
#26468=ADVANCED_FACE ( 'NONE', ( #31991 ), #25090, .F. ) ;
#26487=EDGE_CURVE ( 'NONE', #12228, #42385, #2435, .T. ) ;
#26501=LINE ( 'NONE', #33368, #14851 ) ;
#26516=CARTESIAN_POINT ( 'NONE',  ( -24.72409385541305582, -14.90920654474411577, 58.90588235294116970 ) ) ;
#26524=VERTEX_POINT ( 'NONE', #9601 ) ;
#26564=EDGE_CURVE ( 'NONE', #6974, #15234, #12543, .T. ) ;
#26571=VERTEX_POINT ( 'NONE', #38646 ) ;
#26590=VERTEX_POINT ( 'NONE', #24120 ) ;
#26615=PLANE ( 'NONE',  #38338 ) ;
#26623=ORIENTED_EDGE ( 'NONE', *, *, #25012, .T. ) ;
#26631=EDGE_CURVE ( 'NONE', #6712, #1863, #1455, .T. ) ;
#26660=VECTOR ( 'NONE', #18012, 1000.000000000000000 ) ;
#26673=EDGE_CURVE ( 'NONE', #17004, #22618, #40342, .T. ) ;
#26680=CARTESIAN_POINT ( 'NONE',  ( -50.42609385541305755, -14.80920654474419074, 65.04705882352939739 ) ) ;
#26698=CARTESIAN_POINT ( 'NONE',  ( -42.81012326717776517, -14.90920654474412643, 59.91176470588234793 ) ) ;
#26721=DIRECTION ( 'NONE',  ( -1.000000000000000000, -2.866981220435666553E-17, 0.000000000000000000 ) ) ;
#26725=CARTESIAN_POINT ( 'NONE',  ( -24.72409385541305582, -14.80920654474412679, 59.01176470588234224 ) ) ;
#26736=EDGE_CURVE ( 'NONE', #40267, #31211, #32476, .T. ) ;
#26740=EDGE_CURVE ( 'NONE', #46626, #40821, #29265, .T. ) ;
#26748=EDGE_LOOP ( 'NONE', ( #1332, #25796, #40060, #24928 ) ) ;
#26750=EDGE_CURVE ( 'NONE', #9308, #41453, #28303, .T. ) ;
#26797=CARTESIAN_POINT ( 'NONE',  ( -50.42609385541305755, -14.80920654474411613, 58.90588235294116970 ) ) ;
#26912=ORIENTED_EDGE ( 'NONE', *, *, #432, .F. ) ;
#26919=LINE ( 'NONE', #7730, #25233 ) ;
#26930=CARTESIAN_POINT ( 'NONE',  ( -43.17409385541305511, -14.80920654474410547, 56.99999999999998579 ) ) ;
#27009=EDGE_CURVE ( 'NONE', #29759, #35234, #13622, .T. ) ;
#27016=EDGE_LOOP ( 'NONE', ( #30072, #25716, #7160, #10337, #4875, #10129, #42077, #42762, #24150, #15080, #22848, #44756, #30622, #38296, #14088, #41686, #32068, #4074, #38703, #42255, #26078, #41192, #21059, #41081, #26623, #10677, #35887, #47483, #38330, #31388, #46826, #23915, #22893, #16538, #46198, #48002, #13654, #31175, #8630, #665, #30954, #22041, #13079, #44538, #21830, #16440, #32524, #25587, #31332, #5224, #26912, #35916, #13106, #5370, #4891, #35485, #20641, #35192, #30004, #39147, #40743, #38016, #28041, #47947, #10898, #16157, #44840, #17922, #9314, #3312, #12557, #13544 ) ) ;
#27036=LINE ( 'NONE', #23597, #5222 ) ;
#27041=ORIENTED_EDGE ( 'NONE', *, *, #3169, .T. ) ;
#27042=CARTESIAN_POINT ( 'NONE',  ( -50.42609385541305755, -14.90920654474427565, 73.09411764705880898 ) ) ;
#27043=EDGE_CURVE ( 'NONE', #47792, #11232, #9229, .T. ) ;
#27060=DIRECTION ( 'NONE',  ( -2.866981220435666553E-17, 1.000000000000000000, 1.190614954331866791E-16 ) ) ;
#27084=VERTEX_POINT ( 'NONE', #14814 ) ;
#27091=CARTESIAN_POINT ( 'NONE',  ( -42.67115267894246955, -14.80920654474410547, 61.02352941176469869 ) ) ;
#27094=DIRECTION ( 'NONE',  ( -3.413470714839332458E-33, 1.190614954331866791E-16, -1.000000000000000000 ) ) ;
#27116=CARTESIAN_POINT ( 'NONE',  ( -24.72409385541305582, -14.80920654474410547, 56.99999999999998579 ) ) ;
#27124=CARTESIAN_POINT ( 'NONE',  ( -24.72409385541305582, -14.80920654474423159, 69.97058823529410176 ) ) ;
#27179=ORIENTED_EDGE ( 'NONE', *, *, #40353, .F. ) ;
#27193=EDGE_CURVE ( 'NONE', #29528, #38066, #40701, .T. ) ;
#27207=EDGE_LOOP ( 'NONE', ( #6037, #5667, #32207, #33970 ) ) ;
#27218=DIRECTION ( 'NONE',  ( 1.000000000000000000, 2.866981220435666553E-17, 0.000000000000000000 ) ) ;
#27227=CARTESIAN_POINT ( 'NONE',  ( -24.72409385541305582, -14.80920654474422271, 68.06470588235292496 ) ) ;
#27274=LINE ( 'NONE', #42786, #36952 ) ;
#27298=CARTESIAN_POINT ( 'NONE',  ( -50.42609385541305755, -14.90920654474421170, 67.95882352941174531 ) ) ;
#27300=VECTOR ( 'NONE', #35793, 1000.000000000000114 ) ;
#27307=ORIENTED_EDGE ( 'NONE', *, *, #43829, .T. ) ;
#27314=DIRECTION ( 'NONE',  ( -1.000000000000000000, -2.866981220435666553E-17, -0.000000000000000000 ) ) ;
#27358=LINE ( 'NONE', #7695, #20411 ) ;
#27464=SHAPE_DEFINITION_REPRESENTATION ( #22879, #41459 ) ;
#27484=EDGE_CURVE ( 'NONE', #1662, #1410, #25620, .T. ) ;
#27488=EDGE_LOOP ( 'NONE', ( #13246, #21982, #26127, #5084 ) ) ;
#27504=FACE_OUTER_BOUND ( 'NONE', #41857, .T. ) ;
#27509=DIRECTION ( 'NONE',  ( 1.000000000000000000, 2.866981220435666553E-17, 0.000000000000000000 ) ) ;
#27520=VERTEX_POINT ( 'NONE', #28605 ) ;
#27541=CARTESIAN_POINT ( 'NONE',  ( -24.72409385541305582, -15.80920654474410725, 65.99999999999998579 ) ) ;
#27558=EDGE_CURVE ( 'NONE', #21562, #47432, #37669, .T. ) ;
#27570=EDGE_CURVE ( 'NONE', #37730, #41749, #37921, .T. ) ;
#27582=VECTOR ( 'NONE', #4030, 1000.000000000000000 ) ;
#27595=EDGE_LOOP ( 'NONE', ( #15834, #11455, #10833, #9646 ) ) ;
#27608=EDGE_CURVE ( 'NONE', #39678, #1919, #18973, .T. ) ;
#27687=LINE ( 'NONE', #16589, #2594 ) ;
#27738=EDGE_LOOP ( 'NONE', ( #2749, #28405, #13723, #20889 ) ) ;
#27791=VECTOR ( 'NONE', #4442, 1000.000000000000000 ) ;
#27813=DIRECTION ( 'NONE',  ( 2.866981220435666553E-17, -1.000000000000000000, -1.190614954331866791E-16 ) ) ;
#27819=EDGE_CURVE ( 'NONE', #11232, #32982, #5897, .T. ) ;
#27827=ORIENTED_EDGE ( 'NONE', *, *, #30733, .T. ) ;
#27838=DIRECTION ( 'NONE',  ( 3.413470714839332458E-33, -1.190614954331866791E-16, 1.000000000000000000 ) ) ;
#27914=CARTESIAN_POINT ( 'NONE',  ( -50.42609385541305755, -14.80920654474427600, 73.09411764705880898 ) ) ;
#27921=VECTOR ( 'NONE', #4595, 1000.000000000000114 ) ;
#27922=CARTESIAN_POINT ( 'NONE',  ( -42.55865267894247239, -14.80920654474414810, 61.92352941176469727 ) ) ;
#27928=CARTESIAN_POINT ( 'NONE',  ( -40.92409385541305511, -14.80920654474410725, 74.99999999999998579 ) ) ;
#27988=DIRECTION ( 'NONE',  ( 2.866981220435666553E-17, -1.000000000000000000, -1.190614954331866791E-16 ) ) ;
#28024=EDGE_CURVE ( 'NONE', #205, #12901, #27274, .T. ) ;
#28031=CARTESIAN_POINT ( 'NONE',  ( -24.72409385541305582, -14.80920654474424225, 70.07647058823528141 ) ) ;
#28041=ORIENTED_EDGE ( 'NONE', *, *, #22728, .F. ) ;
#28051=AXIS2_PLACEMENT_3D ( 'NONE', #45066, #7633, #26327 ) ;
#28067=EDGE_CURVE ( 'NONE', #37829, #19273, #12741, .T. ) ;
#28070=ORIENTED_EDGE ( 'NONE', *, *, #27484, .F. ) ;
#28077=DIRECTION ( 'NONE',  ( -2.866981220435666553E-17, 1.000000000000000000, 1.190614954331866791E-16 ) ) ;
#28119=EDGE_CURVE ( 'NONE', #19883, #12016, #21352, .T. ) ;
#28152=DIRECTION ( 'NONE',  ( 1.000000000000000000, 2.866981220435666553E-17, 0.000000000000000000 ) ) ;
#28169=VECTOR ( 'NONE', #12819, 1000.000000000000000 ) ;
#28191=DIRECTION ( 'NONE',  ( 3.413470714839332458E-33, -1.190614954331866791E-16, 1.000000000000000000 ) ) ;
#28223=DIRECTION ( 'NONE',  ( 2.866981220435666553E-17, -1.000000000000000000, -1.190614954331866791E-16 ) ) ;
#28235=ORIENTED_EDGE ( 'NONE', *, *, #48552, .T. ) ;
#28244=VECTOR ( 'NONE', #16371, 1000.000000000000000 ) ;
#28253=ORIENTED_EDGE ( 'NONE', *, *, #41950, .T. ) ;
#28267=ORIENTED_EDGE ( 'NONE', *, *, #7660, .T. ) ;
#28269=DIRECTION ( 'NONE',  ( 3.413470714839332458E-33, -1.190614954331866791E-16, 1.000000000000000000 ) ) ;
#28303=LINE ( 'NONE', #10550, #36918 ) ;
#28339=EDGE_CURVE ( 'NONE', #45073, #46946, #3587, .T. ) ;
#28343=DIRECTION ( 'NONE',  ( -2.866981220435666553E-17, 1.000000000000000000, 1.190614954331866791E-16 ) ) ;
#28377=CARTESIAN_POINT ( 'NONE',  ( -50.42609385541305755, -14.80920654474413745, 60.91764705882351905 ) ) ;
#28397=DIRECTION ( 'NONE',  ( 2.866981220435666553E-17, -1.000000000000000000, -2.395284034871317367E-16 ) ) ;
#28403=CARTESIAN_POINT ( 'NONE',  ( -42.81012326717776517, -14.80920654474412679, 59.91176470588234793 ) ) ;
#28405=ORIENTED_EDGE ( 'NONE', *, *, #5712, .T. ) ;
#28413=VERTEX_POINT ( 'NONE', #20073 ) ;
#28424=VECTOR ( 'NONE', #3696, 1000.000000000000000 ) ;
#28470=EDGE_LOOP ( 'NONE', ( #22074, #32608, #40385, #37652 ) ) ;
#28488=ORIENTED_EDGE ( 'NONE', *, *, #47661, .T. ) ;
#28510=EDGE_CURVE ( 'NONE', #36768, #19883, #5795, .T. ) ;
#28529=DIRECTION ( 'NONE',  ( 1.000000000000000000, 2.866981220435666553E-17, 0.000000000000000000 ) ) ;
#28532=CARTESIAN_POINT ( 'NONE',  ( -50.42609385541305755, -14.80920654474416942, 63.93529411764704662 ) ) ;
#28560=PLANE ( 'NONE',  #11079 ) ;
#28605=CARTESIAN_POINT ( 'NONE',  ( -42.54541738482483026, -14.80920654474410547, 62.02941176470587692 ) ) ;
#28612=PLANE ( 'NONE',  #13174 ) ;
#28637=DIRECTION ( 'NONE',  ( -2.866981220435666553E-17, 1.000000000000000000, 1.190614954331866791E-16 ) ) ;
#28645=PLANE ( 'NONE',  #12244 ) ;
#28647=DIRECTION ( 'NONE',  ( 2.866981220435666553E-17, -1.000000000000000000, -1.190614954331866791E-16 ) ) ;
#28657=CARTESIAN_POINT ( 'NONE',  ( -50.42609385541305755, -14.90920654474414775, 61.02352941176469869 ) ) ;
#28694=DIRECTION ( 'NONE',  ( 1.000000000000000000, 2.866981220435666553E-17, 0.000000000000000000 ) ) ;
#28712=DIRECTION ( 'NONE',  ( -3.413470714839332458E-33, 1.190614954331866791E-16, -1.000000000000000000 ) ) ;
#28717=ORIENTED_EDGE ( 'NONE', *, *, #5059, .T. ) ;
#28731=CARTESIAN_POINT ( 'NONE',  ( -24.72409385541305582, -14.90920654474420104, 66.05294117647058272 ) ) ;
#28736=EDGE_CURVE ( 'NONE', #33229, #1420, #3414, .T. ) ;
#28743=CARTESIAN_POINT ( 'NONE',  ( -41.55245041649903470, -14.90920654474425433, 69.97314751131220589 ) ) ;
#28758=CARTESIAN_POINT ( 'NONE',  ( -24.72409385541305582, -14.80920654474411613, 58.00588235294116402 ) ) ;
#28769=EDGE_CURVE ( 'NONE', #30155, #10544, #2451, .T. ) ;
#28777=ADVANCED_FACE ( 'NONE', ( #43831 ), #28560, .T. ) ;
#28778=CARTESIAN_POINT ( 'NONE',  ( -41.30129973776600139, -14.80920654474425291, 71.98235294117645822 ) ) ;
#28793=DIRECTION ( 'NONE',  ( 1.000000000000000000, 2.866981220435666553E-17, 0.000000000000000000 ) ) ;
#28868=LINE ( 'NONE', #47824, #33776 ) ;
#28886=CARTESIAN_POINT ( 'NONE',  ( -24.72409385541305582, -14.90920654474417972, 64.04117647058822627 ) ) ;
#28951=ORIENTED_EDGE ( 'NONE', *, *, #1620, .T. ) ;
#28984=EDGE_CURVE ( 'NONE', #33229, #30155, #8107, .T. ) ;
#29000=VECTOR ( 'NONE', #11594, 1000.000000000000000 ) ;
#29026=CARTESIAN_POINT ( 'NONE',  ( -24.72409385541305582, -14.90920654474425255, 71.08235294117645253 ) ) ;
#29031=AXIS2_PLACEMENT_3D ( 'NONE', #29301, #44568, #33698 ) ;
#29059=DIRECTION ( 'NONE',  ( 1.000000000000000000, 2.866981220435666553E-17, 0.000000000000000000 ) ) ;
#29122=EDGE_CURVE ( 'NONE', #25093, #41531, #33134, .T. ) ;
#29124=DIRECTION ( 'NONE',  ( 3.413470714839332458E-33, -1.190614954331866791E-16, 1.000000000000000000 ) ) ;
#29143=CARTESIAN_POINT ( 'NONE',  ( -42.04765403640853094, -14.90920654474421170, 66.01151855203617913 ) ) ;
#29173=VECTOR ( 'NONE', #34197, 1000.000000000000000 ) ;
#29176=ORIENTED_EDGE ( 'NONE', *, *, #22728, .T. ) ;
#29181=LINE ( 'NONE', #22034, #41279 ) ;
#29190=VECTOR ( 'NONE', #3443, 1000.000000000000000 ) ;
#29230=FACE_OUTER_BOUND ( 'NONE', #9394, .T. ) ;
#29232=VERTEX_POINT ( 'NONE', #48173 ) ;
#29259=DIRECTION ( 'NONE',  ( -2.866981220435666553E-17, 1.000000000000000000, 1.190614954331866791E-16 ) ) ;
#29265=LINE ( 'NONE', #44299, #39302 ) ;
#29288=DIRECTION ( 'NONE',  ( 1.000000000000000000, 2.866981220435666553E-17, 0.000000000000000000 ) ) ;
#29299=ORIENTED_EDGE ( 'NONE', *, *, #21303, .T. ) ;
#29301=CARTESIAN_POINT ( 'NONE',  ( 0.000000000000000000, 0.000000000000000000, 0.000000000000000000 ) ) ;
#29319=ORIENTED_EDGE ( 'NONE', *, *, #26740, .F. ) ;
#29344=ADVANCED_FACE ( 'NONE', ( #4115 ), #34357, .T. ) ;
#29349=ORIENTED_EDGE ( 'NONE', *, *, #20555, .F. ) ;
#29404=ADVANCED_FACE ( 'NONE', ( #30938 ), #45949, .F. ) ;
#29420=CARTESIAN_POINT ( 'NONE',  ( -50.42609385541305755, -14.80920654474415699, 62.02941176470587692 ) ) ;
#29437=CARTESIAN_POINT ( 'NONE',  ( -24.72409385541305582, -14.80920654474411613, 58.90588235294116970 ) ) ;
#29451=LINE ( 'NONE', #40770, #16603 ) ;
#29456=ORIENTED_EDGE ( 'NONE', *, *, #40567, .F. ) ;
#29461=CARTESIAN_POINT ( 'NONE',  ( -24.72409385541305582, -14.80920654474423159, 69.97058823529410176 ) ) ;
#29470=DIRECTION ( 'NONE',  ( -1.000000000000000000, -2.866981220435666553E-17, 0.000000000000000000 ) ) ;
#29482=VERTEX_POINT ( 'NONE', #38794 ) ;
#29527=EDGE_LOOP ( 'NONE', ( #15831, #26148, #38770, #10404 ) ) ;
#29528=VERTEX_POINT ( 'NONE', #18063 ) ;
#29570=EDGE_CURVE ( 'NONE', #43757, #22495, #5804, .T. ) ;
#29574=CARTESIAN_POINT ( 'NONE',  ( -42.05571150247188683, -14.90920654474419038, 65.94705882352940307 ) ) ;
#29584=ORIENTED_EDGE ( 'NONE', *, *, #16130, .T. ) ;
#29588=ORIENTED_EDGE ( 'NONE', *, *, #5333, .F. ) ;
#29611=ORIENTED_EDGE ( 'NONE', *, *, #23870, .F. ) ;
#29645=DIRECTION ( 'NONE',  ( -1.000000000000000000, -2.866981220435666553E-17, -0.000000000000000000 ) ) ;
#29676=AXIS2_PLACEMENT_3D ( 'NONE', #42842, #35433, #4937 ) ;
#29678=EDGE_CURVE ( 'NONE', #24038, #21562, #26445, .T. ) ;
#29698=VERTEX_POINT ( 'NONE', #48121 ) ;
#29730=ORIENTED_EDGE ( 'NONE', *, *, #34909, .F. ) ;
#29758=CARTESIAN_POINT ( 'NONE',  ( -42.29394679658953038, -14.80920654474417830, 64.04117647058822627 ) ) ;
#29759=VERTEX_POINT ( 'NONE', #16069 ) ;
#29771=CARTESIAN_POINT ( 'NONE',  ( -24.72409385541305582, -14.90920654474420104, 66.05294117647058272 ) ) ;
#29784=FACE_OUTER_BOUND ( 'NONE', #45665, .T. ) ;
#29790=AXIS2_PLACEMENT_3D ( 'NONE', #42683, #20021, #12629 ) ;
#29852=DIRECTION ( 'NONE',  ( -1.000000000000000000, -2.866981220435666553E-17, -0.000000000000000000 ) ) ;
#29897=FACE_OUTER_BOUND ( 'NONE', #47236, .T. ) ;
#29900=CARTESIAN_POINT ( 'NONE',  ( -50.42609385541305755, -14.90920654474420104, 66.05294117647058272 ) ) ;
#29913=VERTEX_POINT ( 'NONE', #39950 ) ;
#29934=LINE ( 'NONE', #33853, #41423 ) ;
#29944=MECHANICAL_DESIGN_GEOMETRIC_PRESENTATION_REPRESENTATION('',(#2418),#22107);
#29950=ORIENTED_EDGE ( 'NONE', *, *, #29678, .T. ) ;
#29969=EDGE_LOOP ( 'NONE', ( #34102, #45682, #47413, #1910 ) ) ;
#29979=LINE ( 'NONE', #45016, #41241 ) ;
#30004=ORIENTED_EDGE ( 'NONE', *, *, #27819, .F. ) ;
#30049=DIRECTION ( 'NONE',  ( -1.000000000000000000, -2.866981220435666553E-17, 0.000000000000000000 ) ) ;
#30065=VERTEX_POINT ( 'NONE', #14002 ) ;
#30072=ORIENTED_EDGE ( 'NONE', *, *, #40353, .T. ) ;
#30074=DIRECTION ( 'NONE',  ( -1.000000000000000000, -2.866981220435666553E-17, 0.000000000000000000 ) ) ;
#30088=CARTESIAN_POINT ( 'NONE',  ( -42.68438797306012589, -14.80920654474413745, 60.91764705882351905 ) ) ;
#30106=CARTESIAN_POINT ( 'NONE',  ( -42.79045946627278596, -14.90920654474414775, 60.06907511312216741 ) ) ;
#30108=ORIENTED_EDGE ( 'NONE', *, *, #31913, .F. ) ;
#30155=VERTEX_POINT ( 'NONE', #46266 ) ;
#30156=CARTESIAN_POINT ( 'NONE',  ( -24.72409385541305582, -14.80920654474414810, 61.92352941176469727 ) ) ;
#30161=ORIENTED_EDGE ( 'NONE', *, *, #9765, .F. ) ;
#30176=ORIENTED_EDGE ( 'NONE', *, *, #25609, .T. ) ;
#30219=PLANE ( 'NONE',  #20403 ) ;
#30233=EDGE_LOOP ( 'NONE', ( #38575, #4344, #40370, #34331 ) ) ;
#30253=EDGE_CURVE ( 'NONE', #47529, #47620, #17166, .T. ) ;
#30279=ORIENTED_EDGE ( 'NONE', *, *, #27193, .T. ) ;
#30283=EDGE_LOOP ( 'NONE', ( #32484, #6795, #9395, #17859 ) ) ;
#30315=CARTESIAN_POINT ( 'NONE',  ( -50.42609385541305755, -14.80920654474426534, 72.98823529411762934 ) ) ;
#30319=CARTESIAN_POINT ( 'NONE',  ( -41.67850562011894056, -14.80920654474422271, 68.96470588235293064 ) ) ;
#30323=ORIENTED_EDGE ( 'NONE', *, *, #43485, .F. ) ;
#30357=CARTESIAN_POINT ( 'NONE',  ( -50.42609385541305755, -14.90920654474422236, 68.96470588235293064 ) ) ;
#30358=DIRECTION ( 'NONE',  ( -2.866981220435666553E-17, 1.000000000000000000, 1.190614954331866791E-16 ) ) ;
#30374=EDGE_LOOP ( 'NONE', ( #14547, #7013, #10659, #21165 ) ) ;
#30406=AXIS2_PLACEMENT_3D ( 'NONE', #11030, #13959, #41069 ) ;
#30451=LINE ( 'NONE', #8055, #42839 ) ;
#30465=EDGE_LOOP ( 'NONE', ( #15174, #1241, #31877, #3286 ) ) ;
#30468=DIRECTION ( 'NONE',  ( 1.415640159446835064E-31, -4.937737817590986075E-15, 1.000000000000000000 ) ) ;
#30469=CARTESIAN_POINT ( 'NONE',  ( -24.72409385541305582, -14.80920654474426357, 72.08823529411763786 ) ) ;
#30495=VERTEX_POINT ( 'NONE', #16814 ) ;
#30501=EDGE_CURVE ( 'NONE', #43447, #22665, #20287, .T. ) ;
#30507=VECTOR ( 'NONE', #28529, 1000.000000000000000 ) ;
#30508=AXIS2_PLACEMENT_3D ( 'NONE', #22191, #27094, #11349 ) ;
#30536=( LENGTH_UNIT ( ) NAMED_UNIT ( * ) SI_UNIT ( .MILLI., .METRE. ) );
#30545=CARTESIAN_POINT ( 'NONE',  ( -50.42609385541305755, -14.90920654474427565, 73.09411764705880898 ) ) ;
#30555=FACE_OUTER_BOUND ( 'NONE', #25390, .T. ) ;
#30564=ADVANCED_FACE ( 'NONE', ( #46145 ), #12404, .T. ) ;
#30606=VECTOR ( 'NONE', #4219, 1000.000000000000000 ) ;
#30622=ORIENTED_EDGE ( 'NONE', *, *, #48078, .T. ) ;
#30635=EDGE_CURVE ( 'NONE', #36955, #19273, #43185, .T. ) ;
#30698=LINE ( 'NONE', #42500, #28244 ) ;
#30711=CARTESIAN_POINT ( 'NONE',  ( -40.92409385541305511, -14.80920654474410725, 74.99999999999998579 ) ) ;
#30733=EDGE_CURVE ( 'NONE', #41749, #14925, #4005, .T. ) ;
#30771=ADVANCED_FACE ( 'NONE', ( #42400 ), #38693, .T. ) ;
#30798=CARTESIAN_POINT ( 'NONE',  ( -24.72409385541305582, -14.90920654474422058, 68.06470588235292496 ) ) ;
#30818=FACE_OUTER_BOUND ( 'NONE', #40613, .T. ) ;
#30902=ADVANCED_FACE ( 'NONE', ( #9871 ), #32286, .T. ) ;
#30905=CARTESIAN_POINT ( 'NONE',  ( -24.72409385541305582, -14.80920654474413745, 60.01764705882352047 ) ) ;
#30938=FACE_OUTER_BOUND ( 'NONE', #22240, .T. ) ;
#30954=ORIENTED_EDGE ( 'NONE', *, *, #10376, .T. ) ;
#30957=EDGE_CURVE ( 'NONE', #2110, #41320, #47540, .T. ) ;
#30974=ORIENTED_EDGE ( 'NONE', *, *, #34639, .T. ) ;
#30985=DIRECTION ( 'NONE',  ( 1.000000000000000000, 2.866981220435666553E-17, 0.000000000000000000 ) ) ;
#31014=ORIENTED_EDGE ( 'NONE', *, *, #12454, .T. ) ;
#31056=LINE ( 'NONE', #5199, #2120 ) ;
#31095=EDGE_CURVE ( 'NONE', #17746, #21028, #4191, .T. ) ;
#31115=DIRECTION ( 'NONE',  ( 1.000000000000000000, 2.866981220435666553E-17, 0.000000000000000000 ) ) ;
#31158=EDGE_CURVE ( 'NONE', #19353, #40794, #19193, .T. ) ;
#31160=LINE ( 'NONE', #16368, #16381 ) ;
#31171=CARTESIAN_POINT ( 'NONE',  ( -41.03659385541305937, -14.80920654474428666, 74.09999999999998010 ) ) ;
#31175=ORIENTED_EDGE ( 'NONE', *, *, #5878, .T. ) ;
#31191=CARTESIAN_POINT ( 'NONE',  ( -42.05571150247187973, -14.80920654474419074, 65.94705882352940307 ) ) ;
#31211=VERTEX_POINT ( 'NONE', #16700 ) ;
#31239=EDGE_CURVE ( 'NONE', #21913, #34260, #32692, .T. ) ;
#31256=AXIS2_PLACEMENT_3D ( 'NONE', #14721, #30049, #970 ) ;
#31258=CARTESIAN_POINT ( 'NONE',  ( -50.42609385541305755, -14.90920654474420104, 66.05294117647058272 ) ) ;
#31295=PLANE ( 'NONE',  #9403 ) ;
#31332=ORIENTED_EDGE ( 'NONE', *, *, #29122, .T. ) ;
#31333=DIRECTION ( 'NONE',  ( 1.000000000000000000, 0.000000000000000000, 0.000000000000000000 ) ) ;
#31334=DIRECTION ( 'NONE',  ( 3.413470714839332458E-33, -1.190614954331866791E-16, 1.000000000000000000 ) ) ;
#31344=ORIENTED_EDGE ( 'NONE', *, *, #30501, .F. ) ;
#31388=ORIENTED_EDGE ( 'NONE', *, *, #30957, .T. ) ;
#31480=CARTESIAN_POINT ( 'NONE',  ( -42.79688797306011594, -14.80920654474410547, 60.01764705882351336 ) ) ;
#31495=EDGE_CURVE ( 'NONE', #29913, #1662, #8308, .T. ) ;
#31510=PLANE ( 'NONE',  #29676 ) ;
#31515=LINE ( 'NONE', #11837, #22838 ) ;
#31543=DIRECTION ( 'NONE',  ( -1.000000000000000000, -2.866981220435666553E-17, 0.000000000000000000 ) ) ;
#31545=ORIENTED_EDGE ( 'NONE', *, *, #32916, .T. ) ;
#31562=EDGE_CURVE ( 'NONE', #35234, #39678, #17369, .T. ) ;
#31568=ADVANCED_FACE ( 'NONE', ( #16876 ), #13175, .T. ) ;
#31574=CARTESIAN_POINT ( 'NONE',  ( -41.04982914953070861, -14.80920654474427600, 73.99411764705880046 ) ) ;
#31578=DIRECTION ( 'NONE',  ( -1.000000000000000000, -2.866981220435666553E-17, -0.000000000000000000 ) ) ;
#31621=FACE_OUTER_BOUND ( 'NONE', #2916, .T. ) ;
#31673=ORIENTED_EDGE ( 'NONE', *, *, #4985, .F. ) ;
#31682=CARTESIAN_POINT ( 'NONE',  ( -41.79100562011894482, -14.80920654474410547, 68.06470588235292496 ) ) ;
#31686=VERTEX_POINT ( 'NONE', #3324 ) ;
#31701=DIRECTION ( 'NONE',  ( 2.866981220435666553E-17, -1.000000000000000000, -1.190614954331866791E-16 ) ) ;
#31716=DIRECTION ( 'NONE',  ( 3.413470714839332458E-33, -1.190614954331866791E-16, 1.000000000000000000 ) ) ;
#31723=DIRECTION ( 'NONE',  ( 2.866981220435666553E-17, -1.000000000000000000, -1.190614954331866791E-16 ) ) ;
#31738=PLANE ( 'NONE',  #7591 ) ;
#31781=DIRECTION ( 'NONE',  ( -1.000000000000000000, -2.866981220435666553E-17, 0.000000000000000000 ) ) ;
#31819=CYLINDRICAL_SURFACE ( 'NONE', #8157, 1.250000000000001110 ) ;
#31844=ORIENTED_EDGE ( 'NONE', *, *, #31913, .T. ) ;
#31852=FACE_OUTER_BOUND ( 'NONE', #35240, .T. ) ;
#31871=ORIENTED_EDGE ( 'NONE', *, *, #18591, .F. ) ;
#31877=ORIENTED_EDGE ( 'NONE', *, *, #4136, .T. ) ;
#31893=ORIENTED_EDGE ( 'NONE', *, *, #18161, .F. ) ;
#31897=ORIENTED_EDGE ( 'NONE', *, *, #5113, .T. ) ;
#31913=EDGE_CURVE ( 'NONE', #13312, #6974, #16991, .T. ) ;
#31962=CARTESIAN_POINT ( 'NONE',  ( -24.72409385541305582, -14.90920654474410512, 57.89999999999999147 ) ) ;
#31991=FACE_OUTER_BOUND ( 'NONE', #36037, .T. ) ;
#32006=VECTOR ( 'NONE', #9806, 1000.000000000000000 ) ;
#32034=CIRCLE ( 'NONE', #24942, 1.250000000000001110 ) ;
#32041=DIRECTION ( 'NONE',  ( -2.866981220435666553E-17, 1.000000000000000000, 1.190614954331866791E-16 ) ) ;
#32045=CARTESIAN_POINT ( 'NONE',  ( -24.72409385541305582, -15.80920654474410725, 65.99999999999998579 ) ) ;
#32068=ORIENTED_EDGE ( 'NONE', *, *, #47741, .T. ) ;
#32095=EDGE_CURVE ( 'NONE', #18357, #40783, #23383, .T. ) ;
#32097=CARTESIAN_POINT ( 'NONE',  ( -50.42609385541305755, -14.80920654474420139, 66.95294117647057419 ) ) ;
#32139=ADVANCED_FACE ( 'NONE', ( #38384 ), #34447, .F. ) ;
#32164=CARTESIAN_POINT ( 'NONE',  ( -24.72409385541305582, -14.90920654474415663, 62.02941176470587692 ) ) ;
#32175=CARTESIAN_POINT ( 'NONE',  ( -50.42609385541305755, -14.80920654474423159, 69.97058823529410176 ) ) ;
#32205=DIRECTION ( 'NONE',  ( -3.413470714839332458E-33, 1.190614954331866791E-16, -1.000000000000000000 ) ) ;
#32207=ORIENTED_EDGE ( 'NONE', *, *, #37483, .F. ) ;
#32209=LINE ( 'NONE', #5637, #32006 ) ;
#32215=CARTESIAN_POINT ( 'NONE',  ( -41.41379973776600565, -14.80920654474425291, 71.08235294117645253 ) ) ;
#32269=ORIENTED_EDGE ( 'NONE', *, *, #40556, .F. ) ;
#32286=PLANE ( 'NONE',  #38700 ) ;
#32292=CARTESIAN_POINT ( 'NONE',  ( -42.17145494138591033, -14.90920654474420104, 65.02111131221717244 ) ) ;
#32330=PLANE ( 'NONE',  #13945 ) ;
#32343=DIRECTION ( 'NONE',  ( -3.413470714839332458E-33, 1.190614954331866791E-16, -1.000000000000000000 ) ) ;
#32344=ADVANCED_FACE ( 'NONE', ( #11031 ), #14204, .T. ) ;
#32355=ORIENTED_EDGE ( 'NONE', *, *, #42919, .T. ) ;
#32375=VECTOR ( 'NONE', #24690, 1000.000000000000000 ) ;
#32386=PLANE ( 'NONE',  #22779 ) ;
#32390=CARTESIAN_POINT ( 'NONE',  ( -50.42609385541305755, -14.90920654474422058, 68.06470588235292496 ) ) ;
#32401=FACE_BOUND ( 'NONE', #21239, .T. ) ;
#32420=DIRECTION ( 'NONE',  ( 1.000000000000000000, 2.866981220435666553E-17, 0.000000000000000000 ) ) ;
#32476=LINE ( 'NONE', #28778, #12546 ) ;
#32484=ORIENTED_EDGE ( 'NONE', *, *, #25609, .F. ) ;
#32516=ORIENTED_EDGE ( 'NONE', *, *, #8161, .T. ) ;
#32524=ORIENTED_EDGE ( 'NONE', *, *, #32916, .F. ) ;
#32553=VERTEX_POINT ( 'NONE', #9044 ) ;
#32571=PLANE ( 'NONE',  #41601 ) ;
#32573=DIRECTION ( 'NONE',  ( 2.866981220435666553E-17, -1.000000000000000000, -1.190614954331866791E-16 ) ) ;
#32580=EDGE_CURVE ( 'NONE', #42512, #40794, #47187, .T. ) ;
#32608=ORIENTED_EDGE ( 'NONE', *, *, #38597, .T. ) ;
#32614=CARTESIAN_POINT ( 'NONE',  ( -46.92409385541305511, -15.81020654474410847, 61.49999999999999289 ) ) ;
#32630=CARTESIAN_POINT ( 'NONE',  ( -50.42409385541305511, -14.80920654474410547, 65.99999999999998579 ) ) ;
#32651=CARTESIAN_POINT ( 'NONE',  ( -24.72409385541305582, -14.80920654474411613, 58.90588235294116970 ) ) ;
#32689=DIRECTION ( 'NONE',  ( -1.000000000000000000, -2.866981220435666553E-17, -0.000000000000000000 ) ) ;
#32692=LINE ( 'NONE', #10055, #6363 ) ;
#32726=VECTOR ( 'NONE', #8612, 1000.000000000000000 ) ;
#32760=VECTOR ( 'NONE', #47437, 1000.000000000000000 ) ;
#32834=CARTESIAN_POINT ( 'NONE',  ( -50.42609385541305755, -14.90920654474421170, 67.05882352941175384 ) ) ;
#32890=ADVANCED_FACE ( 'NONE', ( #39253 ), #21276, .F. ) ;
#32893=EDGE_CURVE ( 'NONE', #18335, #47432, #35306, .T. ) ;
#32915=CARTESIAN_POINT ( 'NONE',  ( -50.42609385541305755, -14.80920654474425291, 71.08235294117645253 ) ) ;
#32916=EDGE_CURVE ( 'NONE', #11434, #17028, #27687, .T. ) ;
#32948=LINE ( 'NONE', #14232, #10904 ) ;
#32956=EDGE_LOOP ( 'NONE', ( #20744, #39219, #11473, #9365 ) ) ;
#32970=CARTESIAN_POINT ( 'NONE',  ( -45.67409385541305511, -14.80920654474410547, 61.49999999999999289 ) ) ;
#32979=VECTOR ( 'NONE', #42724, 1000.000000000000000 ) ;
#32982=VERTEX_POINT ( 'NONE', #22236 ) ;
#32984=EDGE_CURVE ( 'NONE', #26571, #9308, #21520, .T. ) ;
#33002=DIRECTION ( 'NONE',  ( 2.866981220435666553E-17, -1.000000000000000000, -1.190614954331866791E-16 ) ) ;
#33003=DIRECTION ( 'NONE',  ( 2.866981220435666553E-17, -1.000000000000000000, -1.190614954331866791E-16 ) ) ;
#33040=ORIENTED_EDGE ( 'NONE', *, *, #7783, .F. ) ;
#33044=CARTESIAN_POINT ( 'NONE',  ( -42.43291738482482600, -14.80920654474415699, 62.92941176470587550 ) ) ;
#33062=LINE ( 'NONE', #14571, #36382 ) ;
#33081=ORIENTED_EDGE ( 'NONE', *, *, #46363, .T. ) ;
#33134=LINE ( 'NONE', #10518, #39408 ) ;
#33147=DIRECTION ( 'NONE',  ( 1.000000000000000000, 2.866981220435666553E-17, 0.000000000000000000 ) ) ;
#33158=DIRECTION ( 'NONE',  ( 2.866981220435666553E-17, -1.000000000000000000, -1.190614954331866791E-16 ) ) ;
#33192=CARTESIAN_POINT ( 'NONE',  ( -41.16232914953070576, -14.80920654474427600, 73.09411764705880898 ) ) ;
#33226=LINE ( 'NONE', #30315, #17049 ) ;
#33229=VERTEX_POINT ( 'NONE', #8268 ) ;
#33232=ORIENTED_EDGE ( 'NONE', *, *, #45296, .T. ) ;
#33250=FACE_OUTER_BOUND ( 'NONE', #15811, .T. ) ;
#33291=ORIENTED_EDGE ( 'NONE', *, *, #29122, .F. ) ;
#33295=ORIENTED_EDGE ( 'NONE', *, *, #27570, .T. ) ;
#33306=EDGE_CURVE ( 'NONE', #19273, #34260, #34588, .T. ) ;
#33349=( NAMED_UNIT ( * ) PLANE_ANGLE_UNIT ( ) SI_UNIT ( $, .RADIAN. ) );
#33368=CARTESIAN_POINT ( 'NONE',  ( -41.42703503188364778, -14.80920654474424225, 70.97647058823527288 ) ) ;
#33478=DIRECTION ( 'NONE',  ( -1.000000000000000000, -2.866981220435666553E-17, 0.000000000000000000 ) ) ;
#33485=CARTESIAN_POINT ( 'NONE',  ( -41.03659385541305937, -14.80920654474410725, 74.09999999999998010 ) ) ;
#33515=EDGE_CURVE ( 'NONE', #21061, #10723, #33062, .T. ) ;
#33521=ORIENTED_EDGE ( 'NONE', *, *, #12560, .F. ) ;
#33522=EDGE_CURVE ( 'NONE', #15022, #10119, #48105, .T. ) ;
#33603=LINE ( 'NONE', #41021, #44659 ) ;
#33651=VECTOR ( 'NONE', #44673, 1000.000000000000114 ) ;
#33684=LINE ( 'NONE', #22387, #15540 ) ;
#33698=DIRECTION ( 'NONE',  ( 1.000000000000000000, 0.000000000000000000, 0.000000000000000000 ) ) ;
#33709=ADVANCED_FACE ( 'NONE', ( #23231 ), #31819, .F. ) ;
#33713=ADVANCED_FACE ( 'NONE', ( #9669 ), #43401, .F. ) ;
#33729=CARTESIAN_POINT ( 'NONE',  ( -24.72409385541305582, -15.80920654474410725, 65.99999999999998579 ) ) ;
#33776=VECTOR ( 'NONE', #10166, 1000.000000000000000 ) ;
#33781=DIRECTION ( 'NONE',  ( 2.866981220435666553E-17, -1.000000000000000000, -1.190614954331866791E-16 ) ) ;
#33782=VECTOR ( 'NONE', #26453, 1000.000000000000000 ) ;
#33803=ORIENTED_EDGE ( 'NONE', *, *, #9009, .F. ) ;
#33813=ADVANCED_FACE ( 'NONE', ( #2017 ), #35258, .T. ) ;
#33845=PRODUCT ( 'Tuned Steel Comb Vibration Teeth', 'Tuned Steel Comb Vibration Teeth', '', ( #45718 ) ) ;
#33853=CARTESIAN_POINT ( 'NONE',  ( -50.42609385541305755, -14.80920654474414810, 61.02352941176469869 ) ) ;
#33868=CARTESIAN_POINT ( 'NONE',  ( -24.72409385541305582, -14.90920654474424190, 70.97647058823527288 ) ) ;
#33938=LINE ( 'NONE', #48721, #17269 ) ;
#33961=( NAMED_UNIT ( * ) PLANE_ANGLE_UNIT ( ) SI_UNIT ( $, .RADIAN. ) );
#33968=LINE ( 'NONE', #738, #28424 ) ;
#33970=ORIENTED_EDGE ( 'NONE', *, *, #7226, .F. ) ;
#33973=ORIENTED_EDGE ( 'NONE', *, *, #41849, .F. ) ;
#34007=EDGE_CURVE ( 'NONE', #39596, #29232, #7671, .T. ) ;
#34020=EDGE_CURVE ( 'NONE', #21415, #16499, #26363, .T. ) ;
#34022=CARTESIAN_POINT ( 'NONE',  ( -24.72409385541305582, -14.80920654474427423, 73.09411764705880898 ) ) ;
#34102=ORIENTED_EDGE ( 'NONE', *, *, #21303, .F. ) ;
#34137=PLANE ( 'NONE',  #10593 ) ;
#34149=ORIENTED_EDGE ( 'NONE', *, *, #9343, .F. ) ;
#34169=ORIENTED_EDGE ( 'NONE', *, *, #47741, .F. ) ;
#34186=DIRECTION ( 'NONE',  ( 1.000000000000000000, 2.866981220435666553E-17, 0.000000000000000000 ) ) ;
#34197=DIRECTION ( 'NONE',  ( 1.000000000000000000, 2.866981220435666553E-17, 0.000000000000000000 ) ) ;
#34220=DIRECTION ( 'NONE',  ( 1.000000000000000000, 0.000000000000000000, 0.000000000000000000 ) ) ;
#34225=DIRECTION ( 'NONE',  ( -3.413470714839332458E-33, 1.190614954331866791E-16, -1.000000000000000000 ) ) ;
#34260=VERTEX_POINT ( 'NONE', #33868 ) ;
#34295=PLANE ( 'NONE',  #41704 ) ;
#34309=ORIENTED_EDGE ( 'NONE', *, *, #36837, .T. ) ;
#34331=ORIENTED_EDGE ( 'NONE', *, *, #36696, .F. ) ;
#34332=AXIS2_PLACEMENT_3D ( 'NONE', #27541, #39100, #1684 ) ;
#34343=VECTOR ( 'NONE', #8035, 1000.000000000000000 ) ;
#34357=PLANE ( 'NONE',  #2429 ) ;
#34376=VECTOR ( 'NONE', #1025, 1000.000000000000114 ) ;
#34407=ORIENTED_EDGE ( 'NONE', *, *, #43829, .F. ) ;
#34447=PLANE ( 'NONE',  #123 ) ;
#34469=DIRECTION ( 'NONE',  ( -2.866981220435666553E-17, 1.000000000000000000, 1.190614954331866791E-16 ) ) ;
#34488=LINE ( 'NONE', #45608, #10839 ) ;
#34494=CARTESIAN_POINT ( 'NONE',  ( -24.72409385541305582, -14.80920654474411613, 58.00588235294116402 ) ) ;
#34517=VECTOR ( 'NONE', #23177, 1000.000000000000000 ) ;
#34546=CARTESIAN_POINT ( 'NONE',  ( -43.17409385541305511, -15.80920654474410725, 56.99999999999998579 ) ) ;
#34588=LINE ( 'NONE', #8041, #4990 ) ;
#34637=EDGE_CURVE ( 'NONE', #23016, #24237, #17809, .T. ) ;
#34639=EDGE_CURVE ( 'NONE', #14925, #4590, #10933, .T. ) ;
#34672=DIRECTION ( 'NONE',  ( -1.000000000000000000, -2.866981220435666553E-17, 0.000000000000000000 ) ) ;
#34691=EDGE_CURVE ( 'NONE', #12901, #7006, #14107, .T. ) ;
#34706=VECTOR ( 'NONE', #38253, 1000.000000000000000 ) ;
#34737=ADVANCED_FACE ( 'NONE', ( #11657 ), #20019, .F. ) ;
#34759=ORIENTED_EDGE ( 'NONE', *, *, #25951, .F. ) ;
#34779=EDGE_LOOP ( 'NONE', ( #24583, #36493, #9461, #47890 ) ) ;
#34789=CARTESIAN_POINT ( 'NONE',  ( -24.72409385541305582, -14.90920654474419038, 65.94705882352940307 ) ) ;
#34825=ORIENTED_EDGE ( 'NONE', *, *, #3104, .T. ) ;
#34854=ORIENTED_EDGE ( 'NONE', *, *, #19032, .T. ) ;
#34863=DIRECTION ( 'NONE',  ( -0.1240347345892086062, 1.145860353393066553E-16, -0.9922778767136676281 ) ) ;
#34899=LINE ( 'NONE', #16666, #24245 ) ;
#34909=EDGE_CURVE ( 'NONE', #12927, #45073, #20984, .T. ) ;
#34918=EDGE_LOOP ( 'NONE', ( #12930, #30279, #45234, #32269 ) ) ;
#34925=DIRECTION ( 'NONE',  ( -2.866981220435666553E-17, 1.000000000000000000, 1.190614954331866791E-16 ) ) ;
#34934=CARTESIAN_POINT ( 'NONE',  ( -40.92409385541305511, -14.80920654474410725, 74.99999999999998579 ) ) ;
#34977=DIRECTION ( 'NONE',  ( -0.1240347345892086062, 1.145860353393066553E-16, -0.9922778767136676281 ) ) ;
#35003=VERTEX_POINT ( 'NONE', #33485 ) ;
#35053=ORIENTED_EDGE ( 'NONE', *, *, #43086, .F. ) ;
#35069=DIRECTION ( 'NONE',  ( 1.000000000000000000, 2.866981220435666553E-17, 0.000000000000000000 ) ) ;
#35070=ORIENTED_EDGE ( 'NONE', *, *, #19799, .F. ) ;
#35106=ORIENTED_EDGE ( 'NONE', *, *, #3104, .F. ) ;
#35117=AXIS2_PLACEMENT_3D ( 'NONE', #32045, #47066, #1269 ) ;
#35192=ORIENTED_EDGE ( 'NONE', *, *, #5333, .T. ) ;
#35204=EDGE_CURVE ( 'NONE', #35946, #15919, #22947, .T. ) ;
#35234=VERTEX_POINT ( 'NONE', #35451 ) ;
#35240=EDGE_LOOP ( 'NONE', ( #47389, #19967, #34825, #30323 ) ) ;
#35258=PLANE ( 'NONE',  #11309 ) ;
#35267=DIRECTION ( 'NONE',  ( 1.000000000000000000, 2.866981220435666553E-17, 0.000000000000000000 ) ) ;
#35284=CARTESIAN_POINT ( 'NONE',  ( -41.67850562011894766, -14.80920654474422271, 68.96470588235293064 ) ) ;
#35298=ORIENTED_EDGE ( 'NONE', *, *, #32095, .F. ) ;
#35306=LINE ( 'NONE', #28657, #1043 ) ;
#35317=DIRECTION ( 'NONE',  ( -2.866981220435666553E-17, 1.000000000000000000, 1.190614954331866791E-16 ) ) ;
#35343=FACE_OUTER_BOUND ( 'NONE', #36449, .T. ) ;
#35354=LINE ( 'NONE', #43244, #24377 ) ;
#35416=DIRECTION ( 'NONE',  ( -2.866981220435666553E-17, 1.000000000000000000, 1.190614954331866791E-16 ) ) ;
#35422=DIRECTION ( 'NONE',  ( -1.000000000000000000, -2.866981220435666553E-17, 0.000000000000000000 ) ) ;
#35426=ORIENTED_EDGE ( 'NONE', *, *, #8985, .T. ) ;
#35433=DIRECTION ( 'NONE',  ( -1.000000000000000000, -2.866981220435666553E-17, 0.000000000000000000 ) ) ;
#35451=CARTESIAN_POINT ( 'NONE',  ( -24.72409385541305582, -14.90920654474415663, 62.92941176470587550 ) ) ;
#35453=DIRECTION ( 'NONE',  ( 0.1240347345892086200, -1.145860353393066553E-16, 0.9922778767136676281 ) ) ;
#35485=ORIENTED_EDGE ( 'NONE', *, *, #3727, .F. ) ;
#35486=CARTESIAN_POINT ( 'NONE',  ( -50.42609385541305755, -14.90920654474416907, 63.93529411764704662 ) ) ;
#35539=CARTESIAN_POINT ( 'NONE',  ( -41.30129973776600139, -14.80920654474425291, 71.98235294117645822 ) ) ;
#35544=ORIENTED_EDGE ( 'NONE', *, *, #12988, .T. ) ;
#35611=LINE ( 'NONE', #27227, #15321 ) ;
#35635=CARTESIAN_POINT ( 'NONE',  ( -50.42609385541305755, -14.80920654474422271, 68.96470588235293064 ) ) ;
#35663=DIRECTION ( 'NONE',  ( 1.000000000000000000, 2.866981220435666553E-17, 0.000000000000000000 ) ) ;
#35686=DIRECTION ( 'NONE',  ( -2.866981220435666553E-17, 1.000000000000000000, 1.190614954331866791E-16 ) ) ;
#35696=DIRECTION ( 'NONE',  ( -2.866981220435666553E-17, 1.000000000000000000, 1.190614954331866791E-16 ) ) ;
#35724=DIRECTION ( 'NONE',  ( 2.866981220435666553E-17, -1.000000000000000000, -1.190614954331866791E-16 ) ) ;
#35735=CARTESIAN_POINT ( 'NONE',  ( -50.42609385541305755, -14.80920654474419074, 65.94705882352940307 ) ) ;
#35745=VECTOR ( 'NONE', #27060, 1000.000000000000000 ) ;
#35765=PLANE ( 'NONE',  #25147 ) ;
#35767=ORIENTED_EDGE ( 'NONE', *, *, #19032, .F. ) ;
#35768=DIRECTION ( 'NONE',  ( 2.866981220435666553E-17, -1.000000000000000000, -1.190614954331866791E-16 ) ) ;
#35793=DIRECTION ( 'NONE',  ( -0.1240347345892086200, 1.145860353393066553E-16, -0.9922778767136676281 ) ) ;
#35812=ORIENTED_EDGE ( 'NONE', *, *, #45538, .F. ) ;
#35826=CARTESIAN_POINT ( 'NONE',  ( -40.92409385541305511, -14.80920654474410725, 74.99999999999998579 ) ) ;
#35827=DIRECTION ( 'NONE',  ( 2.866981220435666553E-17, -1.000000000000000000, -1.190614954331866791E-16 ) ) ;
#35829=ORIENTED_EDGE ( 'NONE', *, *, #37047, .F. ) ;
#35838=CARTESIAN_POINT ( 'NONE',  ( -24.72409385541305582, -14.90920654474416907, 63.93529411764704662 ) ) ;
#35840=DIRECTION ( 'NONE',  ( -2.866981220435666553E-17, 1.000000000000000000, 1.190614954331866791E-16 ) ) ;
#35853=ORIENTED_EDGE ( 'NONE', *, *, #37854, .F. ) ;
#35857=LINE ( 'NONE', #17136, #42339 ) ;
#35867=DIRECTION ( 'NONE',  ( -0.1240347345892086200, 1.145860353393066553E-16, -0.9922778767136676281 ) ) ;
#35887=ORIENTED_EDGE ( 'NONE', *, *, #14611, .F. ) ;
#35906=SURFACE_STYLE_FILL_AREA ( #16946 ) ;
#35916=ORIENTED_EDGE ( 'NONE', *, *, #19149, .F. ) ;
#35927=CARTESIAN_POINT ( 'NONE',  ( -24.72409385541305582, -14.80920654474418896, 65.94705882352940307 ) ) ;
#35946=VERTEX_POINT ( 'NONE', #47104 ) ;
#35948=ADVANCED_FACE ( 'NONE', ( #24705 ), #5975, .T. ) ;
#35975=ORIENTED_EDGE ( 'NONE', *, *, #12330, .F. ) ;
#36037=EDGE_LOOP ( 'NONE', ( #45745, #12551, #2007, #7509 ) ) ;
#36051=AXIS2_PLACEMENT_3D ( 'NONE', #7188, #10395, #33003 ) ;
#36058=DIRECTION ( 'NONE',  ( 2.866981220435666553E-17, -1.000000000000000000, -1.190614954331866791E-16 ) ) ;
#36061=VECTOR ( 'NONE', #35867, 1000.000000000000114 ) ;
#36069=PLANE ( 'NONE',  #8671 ) ;
#36078=EDGE_LOOP ( 'NONE', ( #19559, #316, #13507, #11834 ) ) ;
#36102=PLANE ( 'NONE',  #9161 ) ;
#36147=DIRECTION ( 'NONE',  ( -0.1240347345892086200, 2.341226830773357975E-16, -0.9922778767136676281 ) ) ;
#36193=ADVANCED_FACE ( 'NONE', ( #20465 ), #46801, .F. ) ;
#36203=FACE_OUTER_BOUND ( 'NONE', #7189, .T. ) ;
#36205=EDGE_LOOP ( 'NONE', ( #14939, #17728, #4352, #20638 ) ) ;
#36323=EDGE_CURVE ( 'NONE', #42514, #1374, #45989, .T. ) ;
#36324=ORIENTED_EDGE ( 'NONE', *, *, #9343, .T. ) ;
#36335=CARTESIAN_POINT ( 'NONE',  ( -50.42609385541305755, -14.80920654474416764, 63.03529411764704804 ) ) ;
#36355=LINE ( 'NONE', #17148, #3814 ) ;
#36382=VECTOR ( 'NONE', #10207, 1000.000000000000114 ) ;
#36392=EDGE_CURVE ( 'NONE', #12228, #24038, #13188, .T. ) ;
#36414=VERTEX_POINT ( 'NONE', #32651 ) ;
#36443=EDGE_CURVE ( 'NONE', #4590, #1374, #35611, .T. ) ;
#36449=EDGE_LOOP ( 'NONE', ( #21431, #11540, #4260, #20634 ) ) ;
#36456=DIRECTION ( 'NONE',  ( 1.000000000000000000, 2.866981220435666553E-17, 0.000000000000000000 ) ) ;
#36461=EDGE_LOOP ( 'NONE', ( #17732, #44579, #2455, #42673 ) ) ;
#36464=EDGE_CURVE ( 'NONE', #43757, #12901, #30451, .T. ) ;
#36471=ORIENTED_EDGE ( 'NONE', *, *, #38880, .T. ) ;
#36488=LINE ( 'NONE', #14071, #42129 ) ;
#36493=ORIENTED_EDGE ( 'NONE', *, *, #16093, .T. ) ;
#36524=DIRECTION ( 'NONE',  ( -3.413470714839332458E-33, 1.190614954331866791E-16, -1.000000000000000000 ) ) ;
#36554=EDGE_LOOP ( 'NONE', ( #7629, #252, #27179, #36324 ) ) ;
#36592=CARTESIAN_POINT ( 'NONE',  ( -41.80424091423659405, -14.90920654474421170, 67.95882352941174531 ) ) ;
#36629=CARTESIAN_POINT ( 'NONE',  ( -41.53953503188365204, -14.80920654474410725, 70.07647058823528141 ) ) ;
#36630=ORIENTED_EDGE ( 'NONE', *, *, #1641, .F. ) ;
#36636=CARTESIAN_POINT ( 'NONE',  ( -50.42609385541305755, -14.90920654474415841, 62.02941176470587692 ) ) ;
#36684=FACE_OUTER_BOUND ( 'NONE', #25788, .T. ) ;
#36696=EDGE_CURVE ( 'NONE', #24126, #41453, #40477, .T. ) ;
#36768=VERTEX_POINT ( 'NONE', #3238 ) ;
#36776=DIRECTION ( 'NONE',  ( -2.866981220435666553E-17, 1.000000000000000000, 1.190614954331866791E-16 ) ) ;
#36785=VECTOR ( 'NONE', #12863, 1000.000000000000000 ) ;
#36821=CARTESIAN_POINT ( 'NONE',  ( -45.92409385541305511, -15.80920654474410725, 70.50000000000000000 ) ) ;
#36837=EDGE_CURVE ( 'NONE', #1662, #15022, #3476, .T. ) ;
#36846=LINE ( 'NONE', #32915, #30507 ) ;
#36918=VECTOR ( 'NONE', #40571, 1000.000000000000000 ) ;
#36952=VECTOR ( 'NONE', #42300, 1000.000000000000000 ) ;
#36955=VERTEX_POINT ( 'NONE', #16498 ) ;
#36961=DIRECTION ( 'NONE',  ( 3.413470714839332458E-33, -1.190614954331866791E-16, 1.000000000000000000 ) ) ;
#36963=LINE ( 'NONE', #10167, #43614 ) ;
#36976=ORIENTED_EDGE ( 'NONE', *, *, #45538, .T. ) ;
#37022=DIRECTION ( 'NONE',  ( -0.1240347345892086062, 1.145860353393066553E-16, -0.9922778767136676281 ) ) ;
#37026=ORIENTED_EDGE ( 'NONE', *, *, #45902, .T. ) ;
#37031=EDGE_CURVE ( 'NONE', #35003, #205, #44322, .T. ) ;
#37047=EDGE_CURVE ( 'NONE', #19438, #5607, #19279, .T. ) ;
#37057=SURFACE_SIDE_STYLE ('',( #35906 ) ) ;
#37074=DIRECTION ( 'NONE',  ( -0.1240347345892086200, 1.145860353393066553E-16, -0.9922778767136676281 ) ) ;
#37093=CARTESIAN_POINT ( 'NONE',  ( -50.42609385541305755, -14.80920654474412679, 59.91176470588234793 ) ) ;
#37100=DIRECTION ( 'NONE',  ( 2.866981220435666553E-17, -1.000000000000000000, -1.190614954331866791E-16 ) ) ;
#37101=CARTESIAN_POINT ( 'NONE',  ( -42.93585856129541156, -14.80920654474411613, 58.90588235294116970 ) ) ;
#37147=DIRECTION ( 'NONE',  ( -0.1240347345892086062, 1.145860353393066553E-16, -0.9922778767136676281 ) ) ;
#37178=DIRECTION ( 'NONE',  ( 1.000000000000000000, 2.866981220435666553E-17, 0.000000000000000000 ) ) ;
#37203=FACE_OUTER_BOUND ( 'NONE', #26748, .T. ) ;
#37215=CARTESIAN_POINT ( 'NONE',  ( -50.42609385541305755, -14.80920654474420139, 66.05294117647058272 ) ) ;
#37246=DIRECTION ( 'NONE',  ( 2.866981220435666553E-17, -1.000000000000000000, -1.190614954331866791E-16 ) ) ;
#37268=EDGE_CURVE ( 'NONE', #11974, #35003, #1125, .T. ) ;
#37273=ORIENTED_EDGE ( 'NONE', *, *, #14473, .T. ) ;
#37287=VERTEX_POINT ( 'NONE', #3420 ) ;
#37319=ORIENTED_EDGE ( 'NONE', *, *, #28984, .F. ) ;
#37321=VECTOR ( 'NONE', #30985, 1000.000000000000000 ) ;
#37326=ORIENTED_EDGE ( 'NONE', *, *, #13927, .T. ) ;
#37372=DIRECTION ( 'NONE',  ( -2.866981220435666553E-17, 1.000000000000000000, 1.190614954331866791E-16 ) ) ;
#37425=LINE ( 'NONE', #44604, #46543 ) ;
#37449=LINE ( 'NONE', #19007, #5517 ) ;
#37453=DIRECTION ( 'NONE',  ( -0.1240347345892086200, 1.145860353393066553E-16, -0.9922778767136676281 ) ) ;
#37460=ORIENTED_EDGE ( 'NONE', *, *, #31562, .F. ) ;
#37483=EDGE_CURVE ( 'NONE', #21028, #8614, #22028, .T. ) ;
#37525=VECTOR ( 'NONE', #44066, 1000.000000000000000 ) ;
#37530=PLANE ( 'NONE',  #45370 ) ;
#37563=FACE_OUTER_BOUND ( 'NONE', #6018, .T. ) ;
#37581=ORIENTED_EDGE ( 'NONE', *, *, #9570, .F. ) ;
#37592=CARTESIAN_POINT ( 'NONE',  ( -42.55865267894247239, -14.90920654474414775, 61.92352941176469727 ) ) ;
#37643=VECTOR ( 'NONE', #19504, 1000.000000000000000 ) ;
#37652=ORIENTED_EDGE ( 'NONE', *, *, #25727, .T. ) ;
#37664=VECTOR ( 'NONE', #4895, 1000.000000000000000 ) ;
#37669=LINE ( 'NONE', #42113, #15731 ) ;
#37693=VERTEX_POINT ( 'NONE', #26698 ) ;
#37730=VERTEX_POINT ( 'NONE', #35284 ) ;
#37763=ORIENTED_EDGE ( 'NONE', *, *, #25012, .F. ) ;
#37770=ORIENTED_EDGE ( 'NONE', *, *, #26736, .F. ) ;
#37782=LINE ( 'NONE', #23512, #34706 ) ;
#37829=VERTEX_POINT ( 'NONE', #17039 ) ;
#37833=AXIS2_PLACEMENT_3D ( 'NONE', #10368, #17490, #47549 ) ;
#37854=EDGE_CURVE ( 'NONE', #25105, #19438, #36963, .T. ) ;
#37866=LINE ( 'NONE', #29758, #7878 ) ;
#37875=VECTOR ( 'NONE', #33002, 1000.000000000000000 ) ;
#37889=VECTOR ( 'NONE', #43923, 1000.000000000000000 ) ;
#37902=LINE ( 'NONE', #42335, #32726 ) ;
#37921=LINE ( 'NONE', #30319, #19694 ) ;
#37925=CARTESIAN_POINT ( 'NONE',  ( -41.67625132147640699, -14.90920654474424190, 68.98274027149319920 ) ) ;
#37950=FACE_OUTER_BOUND ( 'NONE', #27595, .T. ) ;
#37954=DIRECTION ( 'NONE',  ( 1.000000000000000000, 2.866981220435666553E-17, 0.000000000000000000 ) ) ;
#37956=DIRECTION ( 'NONE',  ( 2.866981220435666553E-17, -1.000000000000000000, -1.190614954331866791E-16 ) ) ;
#37960=FACE_BOUND ( 'NONE', #23914, .T. ) ;
#37961=ORIENTED_EDGE ( 'NONE', *, *, #2705, .T. ) ;
#37968=ADVANCED_FACE ( 'NONE', ( #307 ), #14783, .T. ) ;
#38016=ORIENTED_EDGE ( 'NONE', *, *, #7106, .T. ) ;
#38041=DIRECTION ( 'NONE',  ( 3.413470714839332458E-33, -1.190614954331866791E-16, 1.000000000000000000 ) ) ;
#38053=CARTESIAN_POINT ( 'NONE',  ( -50.42609385541305755, -14.80920654474419074, 65.94705882352940307 ) ) ;
#38066=VERTEX_POINT ( 'NONE', #38926 ) ;
#38097=DIRECTION ( 'NONE',  ( 1.000000000000000000, 2.866981220435666553E-17, 0.000000000000000000 ) ) ;
#38111=EDGE_CURVE ( 'NONE', #7006, #16121, #46806, .T. ) ;
#38126=PLANE ( 'NONE',  #28051 ) ;
#38140=DIRECTION ( 'NONE',  ( 2.866981220435666553E-17, -1.000000000000000000, -1.190614954331866791E-16 ) ) ;
#38141=VECTOR ( 'NONE', #46194, 1000.000000000000000 ) ;
#38184=DIRECTION ( 'NONE',  ( 2.866981220435666553E-17, -1.000000000000000000, -1.190614954331866791E-16 ) ) ;
#38187=LINE ( 'NONE', #30106, #34376 ) ;
#38232=ORIENTED_EDGE ( 'NONE', *, *, #46983, .T. ) ;
#38235=DIRECTION ( 'NONE',  ( 1.000000000000000000, 2.866981220435666553E-17, 0.000000000000000000 ) ) ;
#38249=LINE ( 'NONE', #26462, #24425 ) ;
#38253=DIRECTION ( 'NONE',  ( 1.000000000000000000, 2.866981220435666553E-17, 0.000000000000000000 ) ) ;
#38259=ORIENTED_EDGE ( 'NONE', *, *, #40037, .T. ) ;
#38272=VECTOR ( 'NONE', #34186, 1000.000000000000000 ) ;
#38296=ORIENTED_EDGE ( 'NONE', *, *, #17120, .T. ) ;
#38298=ORIENTED_EDGE ( 'NONE', *, *, #28769, .F. ) ;
#38299=LINE ( 'NONE', #30711, #12351 ) ;
#38330=ORIENTED_EDGE ( 'NONE', *, *, #3886, .T. ) ;
#38337=AXIS2_PLACEMENT_3D ( 'NONE', #24934, #14300, #10409 ) ;
#38338=AXIS2_PLACEMENT_3D ( 'NONE', #41634, #34225, #34469 ) ;
#38340=DIRECTION ( 'NONE',  ( -0.1240347345892086062, 1.145860353393066553E-16, -0.9922778767136676281 ) ) ;
#38350=CARTESIAN_POINT ( 'NONE',  ( -41.80424091423659405, -14.80920654474421205, 67.95882352941174531 ) ) ;
#38376=VECTOR ( 'NONE', #31115, 1000.000000000000000 ) ;
#38380=EDGE_CURVE ( 'NONE', #26170, #42514, #20155, .T. ) ;
#38384=FACE_OUTER_BOUND ( 'NONE', #5760, .T. ) ;
#38409=LINE ( 'NONE', #8392, #29000 ) ;
#38420=ORIENTED_EDGE ( 'NONE', *, *, #28736, .F. ) ;
#38441=VERTEX_POINT ( 'NONE', #2880 ) ;
#38448=AXIS2_PLACEMENT_3D ( 'NONE', #43810, #10069, #47004 ) ;
#38452=EDGE_LOOP ( 'NONE', ( #20965, #16772, #14514, #47424 ) ) ;
#38497=VECTOR ( 'NONE', #16446, 1000.000000000000114 ) ;
#38549=ADVANCED_FACE ( 'NONE', ( #7339 ), #34137, .T. ) ;
#38563=AXIS2_PLACEMENT_3D ( 'NONE', #6837, #33158, #32689 ) ;
#38575=ORIENTED_EDGE ( 'NONE', *, *, #14909, .F. ) ;
#38579=COLOUR_RGB ( '', 0.66274510, 0.83137255, 0.94901961) ;
#38597=EDGE_CURVE ( 'NONE', #24799, #35946, #15172, .T. ) ;
#38603=EDGE_CURVE ( 'NONE', #15059, #47792, #29979, .T. ) ;
#38604=LINE ( 'NONE', #42791, #6930 ) ;
#38612=CARTESIAN_POINT ( 'NONE',  ( -48.17409385541305511, -15.80920654474410725, 61.49999999999999289 ) ) ;
#38646=CARTESIAN_POINT ( 'NONE',  ( -42.18144679658952612, -14.90920654474417972, 64.94117647058821774 ) ) ;
#38688=DIRECTION ( 'NONE',  ( 2.866981220435666553E-17, -1.000000000000000000, -1.190614954331866791E-16 ) ) ;
#38693=PLANE ( 'NONE',  #958 ) ;
#38700=AXIS2_PLACEMENT_3D ( 'NONE', #44108, #2478, #25133 ) ;
#38703=ORIENTED_EDGE ( 'NONE', *, *, #28067, .F. ) ;
#38726=DIRECTION ( 'NONE',  ( -1.000000000000000000, -2.866981220435666553E-17, -0.000000000000000000 ) ) ;
#38733=DIRECTION ( 'NONE',  ( -1.000000000000000000, -2.866981220435666553E-17, 0.000000000000000000 ) ) ;
#38740=DIRECTION ( 'NONE',  ( -3.413470714839332458E-33, 1.190614954331866791E-16, -1.000000000000000000 ) ) ;
#38752=CARTESIAN_POINT ( 'NONE',  ( -42.41968209070717677, -14.90920654474416907, 63.03529411764704804 ) ) ;
#38767=EDGE_LOOP ( 'NONE', ( #33973, #35812 ) ) ;
#38770=ORIENTED_EDGE ( 'NONE', *, *, #40964, .T. ) ;
#38794=CARTESIAN_POINT ( 'NONE',  ( -43.04835856129541583, -14.80920654474410547, 58.00588235294116402 ) ) ;
#38809=EDGE_CURVE ( 'NONE', #32553, #23509, #18509, .T. ) ;
#38828=ORIENTED_EDGE ( 'NONE', *, *, #16130, .F. ) ;
#38870=CARTESIAN_POINT ( 'NONE',  ( -24.72409385541305582, -14.90920654474426321, 72.08823529411763786 ) ) ;
#38880=EDGE_CURVE ( 'NONE', #42696, #37693, #64, .T. ) ;
#38894=EDGE_LOOP ( 'NONE', ( #25212, #5082, #45627, #2362 ) ) ;
#38926=CARTESIAN_POINT ( 'NONE',  ( -41.55277032600130127, -14.90920654474423124, 69.97058823529410176 ) ) ;
#38928=VERTEX_POINT ( 'NONE', #7953 ) ;
#38953=AXIS2_PLACEMENT_3D ( 'NONE', #8415, #41412, #19255 ) ;
#38965=LINE ( 'NONE', #9904, #32375 ) ;
#39036=ORIENTED_EDGE ( 'NONE', *, *, #16424, .F. ) ;
#39100=DIRECTION ( 'NONE',  ( -1.000000000000000000, -2.866981220435666553E-17, 0.000000000000000000 ) ) ;
#39122=EDGE_CURVE ( 'NONE', #24230, #15059, #41831, .T. ) ;
#39147=ORIENTED_EDGE ( 'NONE', *, *, #40964, .F. ) ;
#39164=LINE ( 'NONE', #24652, #45585 ) ;
#39182=LINE ( 'NONE', #35486, #37643 ) ;
#39201=DIRECTION ( 'NONE',  ( -2.866981220435666553E-17, 1.000000000000000000, 1.190614954331866791E-16 ) ) ;
#39219=ORIENTED_EDGE ( 'NONE', *, *, #31495, .T. ) ;
#39253=FACE_OUTER_BOUND ( 'NONE', #22858, .T. ) ;
#39257=ORIENTED_EDGE ( 'NONE', *, *, #10376, .F. ) ;
#39284=CARTESIAN_POINT ( 'NONE',  ( -24.72409385541305582, -15.80920654474410725, 65.99999999999998579 ) ) ;
#39302=VECTOR ( 'NONE', #25563, 1000.000000000000000 ) ;
#39332=VECTOR ( 'NONE', #47927, 1000.000000000000000 ) ;
#39336=VECTOR ( 'NONE', #6675, 1000.000000000000000 ) ;
#39404=CARTESIAN_POINT ( 'NONE',  ( -45.92409385541305511, -14.80920654474410725, 70.50000000000000000 ) ) ;
#39408=VECTOR ( 'NONE', #44024, 1000.000000000000114 ) ;
#39433=CARTESIAN_POINT ( 'NONE',  ( -50.42609385541305755, -14.80920654474421205, 67.05882352941175384 ) ) ;
#39456=DIRECTION ( 'NONE',  ( 1.000000000000000000, 2.866981220435666553E-17, 0.000000000000000000 ) ) ;
#39460=DIRECTION ( 'NONE',  ( 2.866981220435666553E-17, -1.000000000000000000, -1.190614954331866791E-16 ) ) ;
#39461=LINE ( 'NONE', #15642, #6945 ) ;
#39468=DIRECTION ( 'NONE',  ( -1.000000000000000000, -2.866981220435666553E-17, -0.000000000000000000 ) ) ;
#39474=ADVANCED_FACE ( 'NONE', ( #37203 ), #17540, .T. ) ;
#39483=CARTESIAN_POINT ( 'NONE',  ( -24.72409385541305582, -14.80920654474416764, 63.93529411764704662 ) ) ;
#39529=EDGE_CURVE ( 'NONE', #8589, #24799, #11614, .T. ) ;
#39531=ORIENTED_EDGE ( 'NONE', *, *, #45569, .F. ) ;
#39559=CARTESIAN_POINT ( 'NONE',  ( -50.42609385541305755, -14.80920654474414810, 61.92352941176469727 ) ) ;
#39579=CARTESIAN_POINT ( 'NONE',  ( -42.30718209070717961, -14.80920654474416764, 63.93529411764704662 ) ) ;
#39596=VERTEX_POINT ( 'NONE', #27116 ) ;
#39643=EDGE_LOOP ( 'NONE', ( #16511, #4565, #30176, #29319 ) ) ;
#39645=CARTESIAN_POINT ( 'NONE',  ( -42.04247620835423049, -14.80920654474410547, 66.05294117647058272 ) ) ;
#39678=VERTEX_POINT ( 'NONE', #17420 ) ;
#39688=DIRECTION ( 'NONE',  ( -2.866981220435666553E-17, 1.000000000000000000, 1.190614954331866791E-16 ) ) ;
#39693=DIRECTION ( 'NONE',  ( 2.866981220435666553E-17, -1.000000000000000000, -1.190614954331866791E-16 ) ) ;
#39761=ORIENTED_EDGE ( 'NONE', *, *, #47257, .F. ) ;
#39763=LINE ( 'NONE', #21055, #22689 ) ;
#39764=PLANE ( 'NONE',  #44001 ) ;
#39794=ORIENTED_EDGE ( 'NONE', *, *, #2032, .F. ) ;
#39849=EDGE_CURVE ( 'NONE', #31686, #19851, #11991, .T. ) ;
#39892=CARTESIAN_POINT ( 'NONE',  ( -40.92409385541305511, -14.80920654474410725, 74.99999999999998579 ) ) ;
#39896=EDGE_CURVE ( 'NONE', #47432, #15891, #46451, .T. ) ;
#39950=CARTESIAN_POINT ( 'NONE',  ( -42.05571150247188683, -14.80920654474419074, 65.94705882352940307 ) ) ;
#39980=AXIS2_PLACEMENT_3D ( 'NONE', #29900, #10459, #29645 ) ;
#40009=CARTESIAN_POINT ( 'NONE',  ( -50.42609385541305755, -14.90920654474419038, 65.04705882352939739 ) ) ;
#40037=EDGE_CURVE ( 'NONE', #37693, #26590, #29181, .T. ) ;
#40060=ORIENTED_EDGE ( 'NONE', *, *, #48349, .T. ) ;
#40077=EDGE_CURVE ( 'NONE', #43447, #14295, #44225, .T. ) ;
#40111=CARTESIAN_POINT ( 'NONE',  ( -42.55865267894247239, -14.80920654474414810, 61.92352941176469727 ) ) ;
#40128=LINE ( 'NONE', #47517, #10233 ) ;
#40138=CARTESIAN_POINT ( 'NONE',  ( -43.17409385541305511, -15.80920654474410725, 56.99999999999998579 ) ) ;
#40188=FACE_OUTER_BOUND ( 'NONE', #12130, .T. ) ;
#40198=PLANE ( 'NONE',  #38337 ) ;
#40202=CARTESIAN_POINT ( 'NONE',  ( -50.42609385541305755, -14.80920654474418008, 64.94117647058821774 ) ) ;
#40213=CARTESIAN_POINT ( 'NONE',  ( -50.42609385541305755, -14.90920654474412643, 59.01176470588234224 ) ) ;
#40218=CARTESIAN_POINT ( 'NONE',  ( -40.92409385541305511, -14.80920654474410725, 74.99999999999998579 ) ) ;
#40235=DIRECTION ( 'NONE',  ( -2.866981220435666553E-17, 1.000000000000000000, 1.190614954331866791E-16 ) ) ;
#40242=CARTESIAN_POINT ( 'NONE',  ( -41.42703503188364778, -14.90920654474424367, 70.97647058823527288 ) ) ;
#40248=CARTESIAN_POINT ( 'NONE',  ( -24.72409385541305582, -14.80920654474422271, 68.96470588235293064 ) ) ;
#40267=VERTEX_POINT ( 'NONE', #35539 ) ;
#40287=ADVANCED_FACE ( 'NONE', ( #31852 ), #28645, .T. ) ;
#40342=LINE ( 'NONE', #1945, #24371 ) ;
#40353=EDGE_CURVE ( 'NONE', #29232, #43757, #36488, .T. ) ;
#40360=LINE ( 'NONE', #21423, #44826 ) ;
#40370=ORIENTED_EDGE ( 'NONE', *, *, #26750, .T. ) ;
#40385=ORIENTED_EDGE ( 'NONE', *, *, #35204, .T. ) ;
#40386=ORIENTED_EDGE ( 'NONE', *, *, #11206, .T. ) ;
#40413=DIRECTION ( 'NONE',  ( -2.866981220435666553E-17, 1.000000000000000000, 1.190614954331866791E-16 ) ) ;
#40435=CARTESIAN_POINT ( 'NONE',  ( -50.42609385541305755, -14.90920654474412643, 59.01176470588234224 ) ) ;
#40467=VERTEX_POINT ( 'NONE', #4975 ) ;
#40477=LINE ( 'NONE', #2333, #3447 ) ;
#40488=ADVANCED_FACE ( 'NONE', ( #310 ), #42153, .T. ) ;
#40509=PLANE ( 'NONE',  #24454 ) ;
#40513=ORIENTED_EDGE ( 'NONE', *, *, #48695, .F. ) ;
#40541=DIRECTION ( 'NONE',  ( -2.866981220435666553E-17, 1.000000000000000000, 1.190614954331866791E-16 ) ) ;
#40551=DIRECTION ( 'NONE',  ( -0.1240347345892086200, 1.145860353393066553E-16, -0.9922778767136676281 ) ) ;
#40556=EDGE_CURVE ( 'NONE', #40648, #30065, #12108, .T. ) ;
#40557=FACE_OUTER_BOUND ( 'NONE', #36205, .T. ) ;
#40567=EDGE_CURVE ( 'NONE', #30495, #7670, #11621, .T. ) ;
#40571=DIRECTION ( 'NONE',  ( 1.000000000000000000, 2.866981220435666553E-17, 0.000000000000000000 ) ) ;
#40613=EDGE_LOOP ( 'NONE', ( #21935, #41784, #9300, #11250, #23489, #33040, #15632, #33521, #15924, #24858, #13162, #7058, #13341, #31893, #5926, #16989, #40513, #23289, #38828, #36630, #48363, #29611, #5402, #18149, #14815, #8084, #8060, #5242, #33291, #44719, #17798, #34759, #29456, #37581, #16011, #14639, #39257, #13819, #6464, #46901, #47710, #18606, #30108, #5677, #10740, #35767, #8063, #12284, #41213, #5688, #20922, #45207, #37763, #9042, #39036, #6309, #24348, #31344, #18685, #25892, #34169, #31871, #22253, #37770, #25323, #29349, #185, #6896, #19240, #38420, #30161, #14009 ) ) ;
#40648=VERTEX_POINT ( 'NONE', #23929 ) ;
#40659=CARTESIAN_POINT ( 'NONE',  ( -40.92409385541305511, -14.80920654474410725, 74.99999999999998579 ) ) ;
#40693=ORIENTED_EDGE ( 'NONE', *, *, #18591, .T. ) ;
#40694=CARTESIAN_POINT ( 'NONE',  ( -40.92409385541305511, -15.80920654474410725, 74.99999999999998579 ) ) ;
#40701=LINE ( 'NONE', #6980, #18839 ) ;
#40717=LINE ( 'NONE', #6992, #33651 ) ;
#40743=ORIENTED_EDGE ( 'NONE', *, *, #48695, .T. ) ;
#40759=LINE ( 'NONE', #45212, #44653 ) ;
#40770=CARTESIAN_POINT ( 'NONE',  ( -42.79688797306011594, -14.80920654474413745, 60.01764705882352047 ) ) ;
#40783=VERTEX_POINT ( 'NONE', #32970 ) ;
#40793=VERTEX_POINT ( 'NONE', #6894 ) ;
#40794=VERTEX_POINT ( 'NONE', #21910 ) ;
#40821=VERTEX_POINT ( 'NONE', #18204 ) ;
#40840=EDGE_LOOP ( 'NONE', ( #45067, #6181, #46398, #30974 ) ) ;
#40855=DIRECTION ( 'NONE',  ( 1.000000000000000000, 2.866981220435666553E-17, 0.000000000000000000 ) ) ;
#40869=DIRECTION ( 'NONE',  ( 2.866981220435666553E-17, -1.000000000000000000, -1.190614954331866791E-16 ) ) ;
#40881=CARTESIAN_POINT ( 'NONE',  ( -50.42609385541305755, -14.90920654474414775, 61.92352941176469727 ) ) ;
#40885=EDGE_LOOP ( 'NONE', ( #23603, #10441, #23129, #9927 ) ) ;
#40890=ORIENTED_EDGE ( 'NONE', *, *, #26673, .T. ) ;
#40958=CARTESIAN_POINT ( 'NONE',  ( -42.93585856129541156, -14.80920654474411613, 58.90588235294116970 ) ) ;
#40964=EDGE_CURVE ( 'NONE', #48084, #11232, #37902, .T. ) ;
#40965=CARTESIAN_POINT ( 'NONE',  ( -24.72409385541305582, -14.80920654474427423, 73.99411764705880046 ) ) ;
#40971=PLANE ( 'NONE',  #39980 ) ;
#41021=CARTESIAN_POINT ( 'NONE',  ( -24.72409385541305582, -14.80920654474412679, 59.01176470588234224 ) ) ;
#41024=ORIENTED_EDGE ( 'NONE', *, *, #13550, .F. ) ;
#41053=ADVANCED_FACE ( 'NONE', ( #16933 ), #31738, .T. ) ;
#41069=DIRECTION ( 'NONE',  ( -2.866981220435666553E-17, 1.000000000000000000, 1.190614954331866791E-16 ) ) ;
#41081=ORIENTED_EDGE ( 'NONE', *, *, #22285, .F. ) ;
#41179=DIRECTION ( 'NONE',  ( 1.000000000000000000, 2.866981220435666553E-17, 0.000000000000000000 ) ) ;
#41190=LINE ( 'NONE', #8924, #25699 ) ;
#41192=ORIENTED_EDGE ( 'NONE', *, *, #3544, .T. ) ;
#41211=VECTOR ( 'NONE', #37022, 1000.000000000000114 ) ;
#41213=ORIENTED_EDGE ( 'NONE', *, *, #3886, .F. ) ;
#41227=DIRECTION ( 'NONE',  ( 1.000000000000000000, 2.866981220435666553E-17, 0.000000000000000000 ) ) ;
#41232=EDGE_LOOP ( 'NONE', ( #25000, #35426, #31014, #5841 ) ) ;
#41241=VECTOR ( 'NONE', #11261, 1000.000000000000000 ) ;
#41254=ORIENTED_EDGE ( 'NONE', *, *, #44401, .F. ) ;
#41279=VECTOR ( 'NONE', #41227, 1000.000000000000000 ) ;
#41285=CARTESIAN_POINT ( 'NONE',  ( -24.72409385541305582, -14.80920654474410902, 57.89999999999999147 ) ) ;
#41304=DIRECTION ( 'NONE',  ( -3.413470714839332458E-33, 1.190614954331866791E-16, -1.000000000000000000 ) ) ;
#41308=ORIENTED_EDGE ( 'NONE', *, *, #37047, .T. ) ;
#41320=VERTEX_POINT ( 'NONE', #16089 ) ;
#41354=ORIENTED_EDGE ( 'NONE', *, *, #28769, .T. ) ;
#41391=DIRECTION ( 'NONE',  ( -2.866981220435666553E-17, 1.000000000000000000, 1.190614954331866791E-16 ) ) ;
#41412=DIRECTION ( 'NONE',  ( -3.413470714839332458E-33, 1.190614954331866791E-16, -1.000000000000000000 ) ) ;
#41423=VECTOR ( 'NONE', #23042, 1000.000000000000000 ) ;
#41427=CARTESIAN_POINT ( 'NONE',  ( -42.92262326717776943, -14.80920654474410547, 59.01176470588234224 ) ) ;
#41428=CARTESIAN_POINT ( 'NONE',  ( -24.72409385541305582, -14.80920654474427423, 73.99411764705880046 ) ) ;
#41430=DIRECTION ( 'NONE',  ( 2.866981220435666553E-17, -1.000000000000000000, -1.190614954331866791E-16 ) ) ;
#41438=EDGE_CURVE ( 'NONE', #454, #6966, #21270, .T. ) ;
#41453=VERTEX_POINT ( 'NONE', #28886 ) ;
#41459=SHAPE_REPRESENTATION ( 'Tuned Steel Comb Vibration Teeth', ( #29031 ), #42412 ) ;
#41474=DIRECTION ( 'NONE',  ( -0.1240347345892086200, 1.145860353393066553E-16, -0.9922778767136676281 ) ) ;
#41531=VERTEX_POINT ( 'NONE', #33044 ) ;
#41532=ORIENTED_EDGE ( 'NONE', *, *, #28067, .T. ) ;
#41570=LINE ( 'NONE', #7853, #4052 ) ;
#41595=FILL_AREA_STYLE_COLOUR ( '', #38579 ) ;
#41601=AXIS2_PLACEMENT_3D ( 'NONE', #44172, #3005, #35768 ) ;
#41634=CARTESIAN_POINT ( 'NONE',  ( -50.42609385541305755, -14.80920654474422271, 68.06470588235292496 ) ) ;
#41663=CARTESIAN_POINT ( 'NONE',  ( -40.92409385541305511, -14.80920654474410725, 74.99999999999998579 ) ) ;
#41667=VECTOR ( 'NONE', #20826, 1000.000000000000114 ) ;
#41678=VECTOR ( 'NONE', #4065, 1000.000000000000000 ) ;
#41686=ORIENTED_EDGE ( 'NONE', *, *, #14473, .F. ) ;
#41692=CARTESIAN_POINT ( 'NONE',  ( -24.72409385541305582, -14.80920654474414810, 61.92352941176469727 ) ) ;
#41696=DIRECTION ( 'NONE',  ( 1.000000000000000000, 2.866981220435666553E-17, 0.000000000000000000 ) ) ;
#41704=AXIS2_PLACEMENT_3D ( 'NONE', #11414, #7747, #581 ) ;
#41714=VECTOR ( 'NONE', #35827, 1000.000000000000000 ) ;
#41749=VERTEX_POINT ( 'NONE', #20484 ) ;
#41784=ORIENTED_EDGE ( 'NONE', *, *, #37268, .F. ) ;
#41805=ORIENTED_EDGE ( 'NONE', *, *, #36464, .F. ) ;
#41819=AXIS2_PLACEMENT_3D ( 'NONE', #15860, #26721, #19079 ) ;
#41831=LINE ( 'NONE', #42064, #37321 ) ;
#41836=PLANE ( 'NONE',  #20457 ) ;
#41849=EDGE_CURVE ( 'NONE', #24654, #25105, #3663, .T. ) ;
#41857=EDGE_LOOP ( 'NONE', ( #17234, #13391, #9912, #4140 ) ) ;
#41860=CARTESIAN_POINT ( 'NONE',  ( -45.67409385541305511, -15.81020654474410847, 61.49999999999999289 ) ) ;
#41883=FACE_OUTER_BOUND ( 'NONE', #16393, .T. ) ;
#41894=VERTEX_POINT ( 'NONE', #11084 ) ;
#41911=FACE_BOUND ( 'NONE', #38767, .T. ) ;
#41944=LINE ( 'NONE', #8220, #14799 ) ;
#41950=EDGE_CURVE ( 'NONE', #23509, #13312, #7893, .T. ) ;
#41969=CARTESIAN_POINT ( 'NONE',  ( -43.06159385541306506, -14.90920654474410512, 57.89999999999999147 ) ) ;
#41978=ADVANCED_FACE ( 'NONE', ( #18959 ), #261, .T. ) ;
#42043=DIRECTION ( 'NONE',  ( -2.866981220435666553E-17, 1.000000000000000000, 1.190614954331866791E-16 ) ) ;
#42064=CARTESIAN_POINT ( 'NONE',  ( -50.42609385541305755, -14.90920654474413887, 60.91764705882351905 ) ) ;
#42077=ORIENTED_EDGE ( 'NONE', *, *, #43252, .F. ) ;
#42085=LINE ( 'NONE', #32215, #13350 ) ;
#42113=CARTESIAN_POINT ( 'NONE',  ( -24.72409385541305582, -14.90920654474414775, 61.02352941176469869 ) ) ;
#42129=VECTOR ( 'NONE', #2769, 1000.000000000000000 ) ;
#42134=EDGE_LOOP ( 'NONE', ( #34407, #26379, #31897, #45026 ) ) ;
#42153=PLANE ( 'NONE',  #38953 ) ;
#42166=AXIS2_PLACEMENT_3D ( 'NONE', #19656, #22880, #19162 ) ;
#42202=CIRCLE ( 'NONE', #42166, 1.250000000000001110 ) ;
#42204=VECTOR ( 'NONE', #38140, 1000.000000000000000 ) ;
#42224=ADVANCED_FACE ( 'NONE', ( #26054 ), #18153, .T. ) ;
#42233=VECTOR ( 'NONE', #11892, 1000.000000000000000 ) ;
#42255=ORIENTED_EDGE ( 'NONE', *, *, #3169, .F. ) ;
#42277=DIRECTION ( 'NONE',  ( 3.413470714839332458E-33, -1.190614954331866791E-16, 1.000000000000000000 ) ) ;
#42300=DIRECTION ( 'NONE',  ( 3.413470714839332458E-33, -1.190614954331866791E-16, 1.000000000000000000 ) ) ;
#42316=ORIENTED_EDGE ( 'NONE', *, *, #32095, .T. ) ;
#42335=CARTESIAN_POINT ( 'NONE',  ( -50.42609385541305755, -14.80920654474413745, 60.01764705882352047 ) ) ;
#42339=VECTOR ( 'NONE', #43520, 1000.000000000000000 ) ;
#42385=VERTEX_POINT ( 'NONE', #37592 ) ;
#42400=FACE_OUTER_BOUND ( 'NONE', #901, .T. ) ;
#42412=( GEOMETRIC_REPRESENTATION_CONTEXT ( 3 ) GLOBAL_UNCERTAINTY_ASSIGNED_CONTEXT ( ( #43531 ) ) GLOBAL_UNIT_ASSIGNED_CONTEXT ( ( #30536, #33961, #23145 ) ) REPRESENTATION_CONTEXT ( 'NONE', 'WORKASPACE' ) );
#42426=ORIENTED_EDGE ( 'NONE', *, *, #25727, .F. ) ;
#42436=CARTESIAN_POINT ( 'NONE',  ( -42.41968209070717677, -14.80920654474410547, 63.03529411764704804 ) ) ;
#42442=PRODUCT_DEFINITION ( 'UNKNOWN', '', #8597, #12978 ) ;
#42469=FACE_OUTER_BOUND ( 'NONE', #40840, .T. ) ;
#42472=VECTOR ( 'NONE', #22419, 1000.000000000000000 ) ;
#42500=CARTESIAN_POINT ( 'NONE',  ( -43.17409385541305511, -14.80920654474410547, 56.99999999999998579 ) ) ;
#42512=VERTEX_POINT ( 'NONE', #35838 ) ;
#42514=VERTEX_POINT ( 'NONE', #31682 ) ;
#42610=CARTESIAN_POINT ( 'NONE',  ( -50.42409385541305511, -14.80920654474410725, 74.99999999999998579 ) ) ;
#42615=CARTESIAN_POINT ( 'NONE',  ( -50.42609385541305755, -14.90920654474415841, 62.02941176470587692 ) ) ;
#42622=AXIS2_PLACEMENT_3D ( 'NONE', #32097, #29124, #13115 ) ;
#42635=EDGE_LOOP ( 'NONE', ( #22311, #20423, #14209, #12584 ) ) ;
#42643=CARTESIAN_POINT ( 'NONE',  ( -42.67115267894247665, -14.90920654474414775, 61.02352941176469869 ) ) ;
#42673=ORIENTED_EDGE ( 'NONE', *, *, #12330, .T. ) ;
#42683=CARTESIAN_POINT ( 'NONE',  ( -46.92409385541305511, -14.80920654474410547, 61.49999999999999289 ) ) ;
#42686=EDGE_CURVE ( 'NONE', #7144, #13624, #43672, .T. ) ;
#42694=PLANE ( 'NONE',  #21903 ) ;
#42696=VERTEX_POINT ( 'NONE', #28403 ) ;
#42724=DIRECTION ( 'NONE',  ( 2.866981220435666553E-17, -1.000000000000000000, -1.190614954331866791E-16 ) ) ;
#42762=ORIENTED_EDGE ( 'NONE', *, *, #48552, .F. ) ;
#42774=CARTESIAN_POINT ( 'NONE',  ( -41.28806444364835215, -14.80920654474426357, 72.08823529411763786 ) ) ;
#42786=CARTESIAN_POINT ( 'NONE',  ( -24.72409385541305582, -14.80920654474428488, 74.99999999999998579 ) ) ;
#42791=CARTESIAN_POINT ( 'NONE',  ( -24.72409385541305582, -14.80920654474428488, 74.09999999999998010 ) ) ;
#42808=FACE_OUTER_BOUND ( 'NONE', #16357, .T. ) ;
#42816=EDGE_LOOP ( 'NONE', ( #135, #43064, #41308, #23638 ) ) ;
#42820=LINE ( 'NONE', #28031, #18918 ) ;
#42839=VECTOR ( 'NONE', #18601, 1000.000000000000000 ) ;
#42840=ORIENTED_EDGE ( 'NONE', *, *, #1915, .T. ) ;
#42842=CARTESIAN_POINT ( 'NONE',  ( -24.72409385541305582, -15.80920654474410725, 65.99999999999998579 ) ) ;
#42915=PLANE ( 'NONE',  #17178 ) ;
#42919=EDGE_CURVE ( 'NONE', #31686, #48232, #7290, .T. ) ;
#42937=DIRECTION ( 'NONE',  ( -3.413470714839332458E-33, 1.190614954331866791E-16, -1.000000000000000000 ) ) ;
#42952=DIRECTION ( 'NONE',  ( -0.1240347345892086062, 1.145860353393066553E-16, -0.9922778767136676281 ) ) ;
#43002=ADVANCED_FACE ( 'NONE', ( #4319 ), #37530, .F. ) ;
#43039=DIRECTION ( 'NONE',  ( 2.866981220435666553E-17, -1.000000000000000000, -1.190614954331866791E-16 ) ) ;
#43044=AXIS2_PLACEMENT_3D ( 'NONE', #43451, #43695, #40235 ) ;
#43064=ORIENTED_EDGE ( 'NONE', *, *, #37854, .T. ) ;
#43067=AXIS2_PLACEMENT_3D ( 'NONE', #11106, #33478, #23170 ) ;
#43086=EDGE_CURVE ( 'NONE', #18610, #41894, #5285, .T. ) ;
#43148=LINE ( 'NONE', #16540, #18694 ) ;
#43155=EDGE_LOOP ( 'NONE', ( #44221, #28267, #48180, #9472 ) ) ;
#43185=LINE ( 'NONE', #47833, #37889 ) ;
#43244=CARTESIAN_POINT ( 'NONE',  ( -41.91674091423659121, -14.80920654474421205, 67.05882352941175384 ) ) ;
#43252=EDGE_CURVE ( 'NONE', #10544, #6966, #47385, .T. ) ;
#43272=CARTESIAN_POINT ( 'NONE',  ( -50.42409385541305511, -14.80920654474410547, 56.99999999999998579 ) ) ;
#43285=EDGE_LOOP ( 'NONE', ( #28070, #34309, #27307, #19060 ) ) ;
#43292=AXIS2_PLACEMENT_3D ( 'NONE', #9705, #21508, #28647 ) ;
#43322=VECTOR ( 'NONE', #14230, 1000.000000000000000 ) ;
#43365=CARTESIAN_POINT ( 'NONE',  ( -24.72409385541305582, -15.80920654474410725, 65.99999999999998579 ) ) ;
#43401=CYLINDRICAL_SURFACE ( 'NONE', #46674, 1.250000000000001110 ) ;
#43413=FACE_OUTER_BOUND ( 'NONE', #30374, .T. ) ;
#43422=DIRECTION ( 'NONE',  ( -6.867234345585437148E-33, 2.395284034871317367E-16, -1.000000000000000000 ) ) ;
#43447=VERTEX_POINT ( 'NONE', #20004 ) ;
#43451=CARTESIAN_POINT ( 'NONE',  ( -50.42609385541305755, -14.80920654474413745, 60.01764705882352047 ) ) ;
#43464=CARTESIAN_POINT ( 'NONE',  ( -46.92409385541305511, -14.80920654474410547, 61.49999999999999289 ) ) ;
#43466=ORIENTED_EDGE ( 'NONE', *, *, #25951, .T. ) ;
#43485=EDGE_CURVE ( 'NONE', #41320, #10012, #5720, .T. ) ;
#43520=DIRECTION ( 'NONE',  ( -2.866981220435666553E-17, 1.000000000000000000, 1.190614954331866791E-16 ) ) ;
#43531=UNCERTAINTY_MEASURE_WITH_UNIT (LENGTH_MEASURE( 1.000000000000000082E-05 ), #30536, 'distance_accuracy_value', 'NONE');
#43584=VECTOR ( 'NONE', #3790, 1000.000000000000000 ) ;
#43614=VECTOR ( 'NONE', #28637, 1000.000000000000000 ) ;
#43672=LINE ( 'NONE', #20762, #20223 ) ;
#43690=DIRECTION ( 'NONE',  ( -1.000000000000000000, -2.866981220435670867E-17, 3.652049423109068320E-16 ) ) ;
#43695=DIRECTION ( 'NONE',  ( -3.413470714839332458E-33, 1.190614954331866791E-16, -1.000000000000000000 ) ) ;
#43718=ADVANCED_FACE ( 'NONE', ( #15745 ), #31510, .F. ) ;
#43757=VERTEX_POINT ( 'NONE', #42610 ) ;
#43798=VECTOR ( 'NONE', #2368, 1000.000000000000000 ) ;
#43810=CARTESIAN_POINT ( 'NONE',  ( -24.72409385541305582, -15.80920654474410725, 65.99999999999998579 ) ) ;
#43820=VECTOR ( 'NONE', #35663, 1000.000000000000000 ) ;
#43829=EDGE_CURVE ( 'NONE', #15022, #47208, #13734, .T. ) ;
#43831=FACE_OUTER_BOUND ( 'NONE', #42134, .T. ) ;
#43838=DIRECTION ( 'NONE',  ( -1.000000000000000000, -2.866981220435666553E-17, 0.000000000000000000 ) ) ;
#43855=EDGE_CURVE ( 'NONE', #7670, #17028, #17449, .T. ) ;
#43898=PLANE ( 'NONE',  #4659 ) ;
#43923=DIRECTION ( 'NONE',  ( 1.000000000000000000, 2.866981220435666553E-17, 0.000000000000000000 ) ) ;
#43939=EDGE_LOOP ( 'NONE', ( #4231, #16452, #22054, #4807 ) ) ;
#44001=AXIS2_PLACEMENT_3D ( 'NONE', #32390, #36058, #47412 ) ;
#44024=DIRECTION ( 'NONE',  ( -0.1240347345892086062, 1.145860353393066553E-16, -0.9922778767136676281 ) ) ;
#44066=DIRECTION ( 'NONE',  ( 1.000000000000000000, 2.866981220435666553E-17, 0.000000000000000000 ) ) ;
#44079=EDGE_CURVE ( 'NONE', #10723, #36414, #1160, .T. ) ;
#44084=LINE ( 'NONE', #10335, #21993 ) ;
#44094=ORIENTED_EDGE ( 'NONE', *, *, #14909, .T. ) ;
#44108=CARTESIAN_POINT ( 'NONE',  ( -50.42609385541305755, -14.80920654474426534, 72.98823529411762934 ) ) ;
#44139=LINE ( 'NONE', #28377, #25781 ) ;
#44142=LINE ( 'NONE', #10394, #37875 ) ;
#44143=PLANE ( 'NONE',  #36051 ) ;
#44172=CARTESIAN_POINT ( 'NONE',  ( -50.42609385541305755, -14.80920654474413745, 60.91764705882351905 ) ) ;
#44181=ORIENTED_EDGE ( 'NONE', *, *, #43252, .T. ) ;
#44194=LINE ( 'NONE', #29143, #27300 ) ;
#44213=DIRECTION ( 'NONE',  ( -1.000000000000000000, -2.866981220435666553E-17, -0.000000000000000000 ) ) ;
#44221=ORIENTED_EDGE ( 'NONE', *, *, #30635, .F. ) ;
#44225=LINE ( 'NONE', #10704, #20052 ) ;
#44283=EDGE_LOOP ( 'NONE', ( #5954, #12600, #27041, #12762 ) ) ;
#44299=CARTESIAN_POINT ( 'NONE',  ( -24.72409385541305582, -14.80920654474426357, 72.98823529411762934 ) ) ;
#44322=LINE ( 'NONE', #25353, #22339 ) ;
#44340=ADVANCED_FACE ( 'NONE', ( #17621 ), #47200, .F. ) ;
#44385=FACE_OUTER_BOUND ( 'NONE', #2727, .T. ) ;
#44401=EDGE_CURVE ( 'NONE', #28413, #20803, #33603, .T. ) ;
#44502=PLANE ( 'NONE',  #1515 ) ;
#44509=EDGE_CURVE ( 'NONE', #18743, #13624, #43148, .T. ) ;
#44526=ADVANCED_FACE ( 'NONE', ( #9422 ), #19334, .T. ) ;
#44538=ORIENTED_EDGE ( 'NONE', *, *, #2927, .F. ) ;
#44541=CARTESIAN_POINT ( 'NONE',  ( -43.17409385541305511, -14.90920654474410512, 56.99999999999998579 ) ) ;
#44543=DIRECTION ( 'NONE',  ( 1.000000000000000000, 2.866981220435666553E-17, 0.000000000000000000 ) ) ;
#44568=DIRECTION ( 'NONE',  ( 0.000000000000000000, 0.000000000000000000, 1.000000000000000000 ) ) ;
#44575=EDGE_CURVE ( 'NONE', #6612, #47792, #20250, .T. ) ;
#44579=ORIENTED_EDGE ( 'NONE', *, *, #5790, .T. ) ;
#44604=CARTESIAN_POINT ( 'NONE',  ( -48.17409385541305511, -15.81020654474410847, 61.49999999999999289 ) ) ;
#44615=ORIENTED_EDGE ( 'NONE', *, *, #44401, .T. ) ;
#44627=VECTOR ( 'NONE', #28343, 1000.000000000000000 ) ;
#44630=CARTESIAN_POINT ( 'NONE',  ( -42.29394679658953038, -14.90920654474417972, 64.04117647058822627 ) ) ;
#44640=ORIENTED_EDGE ( 'NONE', *, *, #11876, .T. ) ;
#44646=CARTESIAN_POINT ( 'NONE',  ( -24.72409385541305582, -14.80920654474416764, 63.03529411764704804 ) ) ;
#44653=VECTOR ( 'NONE', #48388, 1000.000000000000000 ) ;
#44659=VECTOR ( 'NONE', #44981, 1000.000000000000000 ) ;
#44667=VECTOR ( 'NONE', #37074, 1000.000000000000114 ) ;
#44673=DIRECTION ( 'NONE',  ( -0.1240347345892086062, 1.145860353393066553E-16, -0.9922778767136676281 ) ) ;
#44674=VECTOR ( 'NONE', #11312, 1000.000000000000000 ) ;
#44685=ORIENTED_EDGE ( 'NONE', *, *, #44509, .F. ) ;
#44714=ADVANCED_FACE ( 'NONE', ( #41883 ), #26615, .T. ) ;
#44719=ORIENTED_EDGE ( 'NONE', *, *, #16093, .F. ) ;
#44740=ADVANCED_FACE ( 'NONE', ( #18980 ), #3716, .F. ) ;
#44744=DIRECTION ( 'NONE',  ( 2.866981220435666553E-17, -1.000000000000000000, -1.190614954331866791E-16 ) ) ;
#44756=ORIENTED_EDGE ( 'NONE', *, *, #42686, .F. ) ;
#44812=ADVANCED_FACE ( 'NONE', ( #8156 ), #4443, .T. ) ;
#44825=CARTESIAN_POINT ( 'NONE',  ( -40.92409385541305511, -14.80920654474410725, 74.99999999999998579 ) ) ;
#44826=VECTOR ( 'NONE', #37372, 1000.000000000000000 ) ;
#44840=ORIENTED_EDGE ( 'NONE', *, *, #11876, .F. ) ;
#44879=CARTESIAN_POINT ( 'NONE',  ( -24.72409385541305582, -14.90920654474411577, 58.00588235294116402 ) ) ;
#44885=EDGE_CURVE ( 'NONE', #26170, #4590, #24136, .T. ) ;
#44902=LINE ( 'NONE', #18774, #22129 ) ;
#44905=DIRECTION ( 'NONE',  ( -0.1240347345892086200, 1.145860353393066553E-16, -0.9922778767136676281 ) ) ;
#44975=DIRECTION ( 'NONE',  ( -2.866981220435666553E-17, 1.000000000000000000, 1.190614954331866791E-16 ) ) ;
#44981=DIRECTION ( 'NONE',  ( -2.866981220435666553E-17, 1.000000000000000000, 1.190614954331866791E-16 ) ) ;
#44997=DIRECTION ( 'NONE',  ( 2.866981220435666553E-17, -1.000000000000000000, -1.190614954331866791E-16 ) ) ;
#45011=DIRECTION ( 'NONE',  ( 1.000000000000000000, 0.000000000000000000, 0.000000000000000000 ) ) ;
#45016=CARTESIAN_POINT ( 'NONE',  ( -24.72409385541305582, -14.90920654474413709, 60.01764705882352047 ) ) ;
#45026=ORIENTED_EDGE ( 'NONE', *, *, #1889, .F. ) ;
#45065=CARTESIAN_POINT ( 'NONE',  ( -24.72409385541305582, -14.80920654474419962, 66.05294117647058272 ) ) ;
#45066=CARTESIAN_POINT ( 'NONE',  ( -50.42609385541305755, -14.80920654474410902, 57.89999999999999147 ) ) ;
#45067=ORIENTED_EDGE ( 'NONE', *, *, #36443, .T. ) ;
#45073=VERTEX_POINT ( 'NONE', #29026 ) ;
#45087=EDGE_CURVE ( 'NONE', #17746, #7006, #21644, .T. ) ;
#45097=FACE_OUTER_BOUND ( 'NONE', #36461, .T. ) ;
#45114=CARTESIAN_POINT ( 'NONE',  ( -42.29525584636328972, -14.90920654474419038, 64.03070407239817996 ) ) ;
#45118=LINE ( 'NONE', #40659, #6904 ) ;
#45174=VECTOR ( 'NONE', #24405, 1000.000000000000000 ) ;
#45207=ORIENTED_EDGE ( 'NONE', *, *, #27570, .F. ) ;
#45212=CARTESIAN_POINT ( 'NONE',  ( -24.72409385541305582, -14.90920654474411577, 58.00588235294116402 ) ) ;
#45234=ORIENTED_EDGE ( 'NONE', *, *, #347, .T. ) ;
#45243=VECTOR ( 'NONE', #7947, 1000.000000000000000 ) ;
#45268=ORIENTED_EDGE ( 'NONE', *, *, #21648, .T. ) ;
#45270=VECTOR ( 'NONE', #22968, 1000.000000000000114 ) ;
#45278=ORIENTED_EDGE ( 'NONE', *, *, #16424, .T. ) ;
#45285=CARTESIAN_POINT ( 'NONE',  ( -50.42609385541305755, -14.90920654474428630, 74.99999999999998579 ) ) ;
#45296=EDGE_CURVE ( 'NONE', #16121, #205, #38604, .T. ) ;
#45358=CARTESIAN_POINT ( 'NONE',  ( -50.42609385541305755, -14.90920654474414775, 61.02352941176469869 ) ) ;
#45370=AXIS2_PLACEMENT_3D ( 'NONE', #23520, #15364, #864 ) ;
#45385=LINE ( 'NONE', #15073, #18630 ) ;
#45388=DIRECTION ( 'NONE',  ( 3.413470714839332458E-33, -1.190614954331866791E-16, 1.000000000000000000 ) ) ;
#45396=CARTESIAN_POINT ( 'NONE',  ( -50.42609385541305755, -14.80920654474412679, 59.91176470588234793 ) ) ;
#45400=CARTESIAN_POINT ( 'NONE',  ( -42.43291738482482600, -14.90920654474415841, 62.92941176470587550 ) ) ;
#45416=CARTESIAN_POINT ( 'NONE',  ( -24.72409385541305582, -14.90920654474419038, 65.04705882352939739 ) ) ;
#45423=CARTESIAN_POINT ( 'NONE',  ( -41.04982914953070150, -14.80920654474427600, 73.99411764705880046 ) ) ;
#45470=CARTESIAN_POINT ( 'NONE',  ( -50.42609385541305755, -14.90920654474417972, 64.04117647058822627 ) ) ;
#45472=AXIS2_PLACEMENT_3D ( 'NONE', #40202, #36961, #25651 ) ;
#45524=ORIENTED_EDGE ( 'NONE', *, *, #43086, .T. ) ;
#45538=EDGE_CURVE ( 'NONE', #25105, #24654, #5401, .T. ) ;
#45569=EDGE_CURVE ( 'NONE', #31211, #24237, #31160, .T. ) ;
#45585=VECTOR ( 'NONE', #46328, 1000.000000000000114 ) ;
#45591=CARTESIAN_POINT ( 'NONE',  ( -41.17556444364835500, -14.80920654474426534, 72.98823529411762934 ) ) ;
#45608=CARTESIAN_POINT ( 'NONE',  ( -24.72409385541305582, -14.80920654474427423, 73.99411764705880046 ) ) ;
#45617=LINE ( 'NONE', #19251, #13901 ) ;
#45623=DIRECTION ( 'NONE',  ( -2.866981220435666553E-17, 1.000000000000000000, 1.190614954331866791E-16 ) ) ;
#45627=ORIENTED_EDGE ( 'NONE', *, *, #39529, .T. ) ;
#45655=DIRECTION ( 'NONE',  ( 1.000000000000000000, 2.866981220435666553E-17, 0.000000000000000000 ) ) ;
#45659=VECTOR ( 'NONE', #14193, 1000.000000000000000 ) ;
#45660=DIRECTION ( 'NONE',  ( 2.866981220435666553E-17, -1.000000000000000000, -1.190614954331866791E-16 ) ) ;
#45665=EDGE_LOOP ( 'NONE', ( #23547, #7711, #40386, #25088 ) ) ;
#45670=CARTESIAN_POINT ( 'NONE',  ( -24.72409385541305582, -14.80920654474416764, 63.93529411764704662 ) ) ;
#45679=CARTESIAN_POINT ( 'NONE',  ( -24.72409385541305582, -14.80920654474424225, 70.97647058823527288 ) ) ;
#45682=ORIENTED_EDGE ( 'NONE', *, *, #13893, .T. ) ;
#45718=PRODUCT_CONTEXT ( 'NONE', #15516, 'mechanical' ) ;
#45724=DIRECTION ( 'NONE',  ( 1.000000000000000000, 2.866981220435666553E-17, 0.000000000000000000 ) ) ;
#45733=VECTOR ( 'NONE', #44975, 1000.000000000000000 ) ;
#45745=ORIENTED_EDGE ( 'NONE', *, *, #27043, .T. ) ;
#45786=ORIENTED_EDGE ( 'NONE', *, *, #11731, .F. ) ;
#45805=ORIENTED_EDGE ( 'NONE', *, *, #39896, .F. ) ;
#45808=CARTESIAN_POINT ( 'NONE',  ( -41.03659385541305937, -14.90920654474428630, 74.09999999999998010 ) ) ;
#45820=FACE_OUTER_BOUND ( 'NONE', #46446, .T. ) ;
#45828=EDGE_CURVE ( 'NONE', #45934, #27520, #23454, .T. ) ;
#45832=CARTESIAN_POINT ( 'NONE',  ( -24.72409385541305582, -14.80920654474419962, 66.95294117647057419 ) ) ;
#45857=CARTESIAN_POINT ( 'NONE',  ( -50.42609385541305755, -14.80920654474426534, 72.08823529411763786 ) ) ;
#45902=EDGE_CURVE ( 'NONE', #38928, #42512, #39182, .T. ) ;
#45930=LINE ( 'NONE', #1104, #25003 ) ;
#45934=VERTEX_POINT ( 'NONE', #17493 ) ;
#45949=PLANE ( 'NONE',  #10309 ) ;
#45977=VERTEX_POINT ( 'NONE', #24430 ) ;
#45984=ORIENTED_EDGE ( 'NONE', *, *, #34909, .T. ) ;
#45989=LINE ( 'NONE', #12246, #16094 ) ;
#46045=ORIENTED_EDGE ( 'NONE', *, *, #16695, .T. ) ;
#46084=ADVANCED_FACE ( 'NONE', ( #11091 ), #16, .T. ) ;
#46145=FACE_OUTER_BOUND ( 'NONE', #18086, .T. ) ;
#46149=ORIENTED_EDGE ( 'NONE', *, *, #30253, .F. ) ;
#46194=DIRECTION ( 'NONE',  ( -2.866981220435666553E-17, 1.000000000000000000, 1.190614954331866791E-16 ) ) ;
#46198=ORIENTED_EDGE ( 'NONE', *, *, #38597, .F. ) ;
#46231=LINE ( 'NONE', #19391, #9488 ) ;
#46243=DIRECTION ( 'NONE',  ( -2.866981220435666553E-17, 1.000000000000000000, 1.190614954331866791E-16 ) ) ;
#46266=CARTESIAN_POINT ( 'NONE',  ( -24.72409385541305582, -14.90920654474427565, 73.09411764705880898 ) ) ;
#46267=ORIENTED_EDGE ( 'NONE', *, *, #6200, .F. ) ;
#46276=VECTOR ( 'NONE', #38235, 1000.000000000000000 ) ;
#46298=DIRECTION ( 'NONE',  ( -1.000000000000000000, -2.866981220435666553E-17, -0.000000000000000000 ) ) ;
#46307=ADVANCED_FACE ( 'NONE', ( #43413 ), #42915, .T. ) ;
#46316=CARTESIAN_POINT ( 'NONE',  ( -40.92409385541305511, -14.80920654474410725, 74.99999999999998579 ) ) ;
#46328=DIRECTION ( 'NONE',  ( -0.1240347345892086200, 1.145860353393066553E-16, -0.9922778767136676281 ) ) ;
#46363=EDGE_CURVE ( 'NONE', #40793, #40783, #2253, .T. ) ;
#46364=DIRECTION ( 'NONE',  ( 2.866981220435666553E-17, -1.000000000000000000, -1.190614954331866791E-16 ) ) ;
#46383=LINE ( 'NONE', #45670, #15602 ) ;
#46398=ORIENTED_EDGE ( 'NONE', *, *, #4985, .T. ) ;
#46446=EDGE_LOOP ( 'NONE', ( #39794, #8825, #17874, #37460 ) ) ;
#46451=LINE ( 'NONE', #16389, #1984 ) ;
#46526=VECTOR ( 'NONE', #48601, 1000.000000000000000 ) ;
#46543=VECTOR ( 'NONE', #40413, 1000.000000000000000 ) ;
#46588=EDGE_CURVE ( 'NONE', #2110, #3303, #8166, .T. ) ;
#46610=VERTEX_POINT ( 'NONE', #30088 ) ;
#46619=CARTESIAN_POINT ( 'NONE',  ( -50.42609385541305755, -14.90920654474411577, 58.00588235294116402 ) ) ;
#46626=VERTEX_POINT ( 'NONE', #22948 ) ;
#46666=CARTESIAN_POINT ( 'NONE',  ( -24.72409385541305582, -14.80920654474418896, 65.04705882352939739 ) ) ;
#46667=CARTESIAN_POINT ( 'NONE',  ( -24.72409385541305582, -14.80920654474417830, 64.94117647058821774 ) ) ;
#46668=ORIENTED_EDGE ( 'NONE', *, *, #29678, .F. ) ;
#46674=AXIS2_PLACEMENT_3D ( 'NONE', #23957, #39201, #5235 ) ;
#46687=APPLICATION_CONTEXT ( 'automotive_design' ) ;
#46722=VERTEX_POINT ( 'NONE', #5910 ) ;
#46741=DIRECTION ( 'NONE',  ( 2.866981220435666553E-17, -1.000000000000000000, -1.190614954331866791E-16 ) ) ;
#46750=CARTESIAN_POINT ( 'NONE',  ( -24.72409385541305582, -14.80920654474410902, 57.89999999999999147 ) ) ;
#46758=DIRECTION ( 'NONE',  ( 3.413470714839332458E-33, -1.190614954331866791E-16, 1.000000000000000000 ) ) ;
#46782=ADVANCED_FACE ( 'NONE', ( #47521 ), #21427, .F. ) ;
#46801=PLANE ( 'NONE',  #48340 ) ;
#46806=LINE ( 'NONE', #9385, #45174 ) ;
#46820=FACE_OUTER_BOUND ( 'NONE', #4029, .T. ) ;
#46826=ORIENTED_EDGE ( 'NONE', *, *, #23275, .F. ) ;
#46865=VERTEX_POINT ( 'NONE', #19602 ) ;
#46899=CARTESIAN_POINT ( 'NONE',  ( -42.92262326717776943, -14.90920654474412643, 59.01176470588234224 ) ) ;
#46901=ORIENTED_EDGE ( 'NONE', *, *, #31495, .F. ) ;
#46906=AXIS2_PLACEMENT_3D ( 'NONE', #30545, #15237, #27314 ) ;
#46912=DIRECTION ( 'NONE',  ( 2.866981220435666553E-17, -1.000000000000000000, -1.190614954331866791E-16 ) ) ;
#46946=VERTEX_POINT ( 'NONE', #896 ) ;
#46983=EDGE_CURVE ( 'NONE', #40794, #11434, #10227, .T. ) ;
#46999=ADVANCED_FACE ( 'NONE', ( #35343 ), #39764, .T. ) ;
#47004=DIRECTION ( 'NONE',  ( -2.866981220435666553E-17, 1.000000000000000000, 1.190614954331866791E-16 ) ) ;
#47066=DIRECTION ( 'NONE',  ( -1.000000000000000000, -2.866981220435666553E-17, 0.000000000000000000 ) ) ;
#47100=FACE_OUTER_BOUND ( 'NONE', #9725, .T. ) ;
#47101=ORIENTED_EDGE ( 'NONE', *, *, #38111, .T. ) ;
#47104=CARTESIAN_POINT ( 'NONE',  ( -24.72409385541305582, -14.80920654474419962, 66.95294117647057419 ) ) ;
#47142=EDGE_LOOP ( 'NONE', ( #8633, #14233 ) ) ;
#47150=ORIENTED_EDGE ( 'NONE', *, *, #18161, .T. ) ;
#47183=AXIS2_PLACEMENT_3D ( 'NONE', #37093, #18136, #6593 ) ;
#47187=LINE ( 'NONE', #13182, #8037 ) ;
#47200=PLANE ( 'NONE',  #15529 ) ;
#47208=VERTEX_POINT ( 'NONE', #45416 ) ;
#47236=EDGE_LOOP ( 'NONE', ( #35106, #13628, #14450, #4734 ) ) ;
#47238=EDGE_CURVE ( 'NONE', #22618, #41894, #19801, .T. ) ;
#47251=CARTESIAN_POINT ( 'NONE',  ( -24.72409385541305582, -14.80920654474423159, 69.07058823529411029 ) ) ;
#47257=EDGE_CURVE ( 'NONE', #37730, #29698, #1304, .T. ) ;
#47260=( NAMED_UNIT ( * ) SI_UNIT ( $, .STERADIAN. ) SOLID_ANGLE_UNIT ( ) );
#47284=VECTOR ( 'NONE', #10367, 1000.000000000000114 ) ;
#47298=CARTESIAN_POINT ( 'NONE',  ( -45.67409385541305511, -15.80920654474410725, 61.49999999999999289 ) ) ;
#47305=VECTOR ( 'NONE', #6661, 1000.000000000000000 ) ;
#47314=CARTESIAN_POINT ( 'NONE',  ( -50.42609385541305755, -14.90920654474426499, 72.08823529411763786 ) ) ;
#47365=DIRECTION ( 'NONE',  ( -2.866981220435666553E-17, 1.000000000000000000, 1.190614954331866791E-16 ) ) ;
#47385=LINE ( 'NONE', #41428, #42233 ) ;
#47389=ORIENTED_EDGE ( 'NONE', *, *, #30957, .F. ) ;
#47396=LINE ( 'NONE', #46667, #1679 ) ;
#47412=DIRECTION ( 'NONE',  ( -1.000000000000000000, -2.866981220435666553E-17, -0.000000000000000000 ) ) ;
#47413=ORIENTED_EDGE ( 'NONE', *, *, #32893, .T. ) ;
#47424=ORIENTED_EDGE ( 'NONE', *, *, #18017, .T. ) ;
#47432=VERTEX_POINT ( 'NONE', #9692 ) ;
#47437=DIRECTION ( 'NONE',  ( 1.000000000000000000, 2.866981220435666553E-17, 0.000000000000000000 ) ) ;
#47440=LINE ( 'NONE', #36335, #23427 ) ;
#47448=CARTESIAN_POINT ( 'NONE',  ( -24.72409385541305582, -14.80920654474423159, 69.07058823529411029 ) ) ;
#47453=EDGE_LOOP ( 'NONE', ( #8335, #2398, #32355, #11320 ) ) ;
#47476=ADVANCED_FACE ( 'NONE', ( #44385 ), #25184, .T. ) ;
#47483=ORIENTED_EDGE ( 'NONE', *, *, #36323, .F. ) ;
#47500=CARTESIAN_POINT ( 'NONE',  ( -50.42609385541305755, -14.80920654474416942, 63.93529411764704662 ) ) ;
#47513=AXIS2_PLACEMENT_3D ( 'NONE', #26930, #577, #45660 ) ;
#47517=CARTESIAN_POINT ( 'NONE',  ( -24.72409385541305582, -14.90920654474426321, 72.08823529411763786 ) ) ;
#47521=FACE_OUTER_BOUND ( 'NONE', #14563, .T. ) ;
#47529=VERTEX_POINT ( 'NONE', #44879 ) ;
#47540=LINE ( 'NONE', #6175, #15876 ) ;
#47549=DIRECTION ( 'NONE',  ( -1.000000000000000000, -2.866981220435666553E-17, -0.000000000000000000 ) ) ;
#47615=DIRECTION ( 'NONE',  ( 1.000000000000000000, 2.866981220435666553E-17, 0.000000000000000000 ) ) ;
#47620=VERTEX_POINT ( 'NONE', #34494 ) ;
#47661=EDGE_CURVE ( 'NONE', #19851, #29482, #20209, .T. ) ;
#47665=DIRECTION ( 'NONE',  ( -3.413470714839332458E-33, 1.190614954331866791E-16, -1.000000000000000000 ) ) ;
#47694=LINE ( 'NONE', #28743, #13299 ) ;
#47710=ORIENTED_EDGE ( 'NONE', *, *, #2661, .F. ) ;
#47741=EDGE_CURVE ( 'NONE', #27084, #36955, #24878, .T. ) ;
#47744=DIRECTION ( 'NONE',  ( -2.866981220435666553E-17, 1.000000000000000000, 1.190614954331866791E-16 ) ) ;
#47761=CARTESIAN_POINT ( 'NONE',  ( -24.72409385541305582, -14.90920654474413709, 60.01764705882352047 ) ) ;
#47792=VERTEX_POINT ( 'NONE', #47761 ) ;
#47811=CARTESIAN_POINT ( 'NONE',  ( -43.06159385541306506, -14.80920654474410547, 57.89999999999999147 ) ) ;
#47824=CARTESIAN_POINT ( 'NONE',  ( -42.92262326717776943, -14.80920654474412679, 59.01176470588234224 ) ) ;
#47825=VECTOR ( 'NONE', #10757, 1000.000000000000114 ) ;
#47833=CARTESIAN_POINT ( 'NONE',  ( -50.42609385541305755, -14.80920654474424225, 70.97647058823527288 ) ) ;
#47845=VECTOR ( 'NONE', #37453, 1000.000000000000114 ) ;
#47854=VECTOR ( 'NONE', #45655, 1000.000000000000000 ) ;
#47890=ORIENTED_EDGE ( 'NONE', *, *, #46983, .F. ) ;
#47913=AXIS2_PLACEMENT_3D ( 'NONE', #35635, #31716, #43039 ) ;
#47915=VERTEX_POINT ( 'NONE', #721 ) ;
#47927=DIRECTION ( 'NONE',  ( -2.866981220435666553E-17, 1.000000000000000000, 1.190614954331866791E-16 ) ) ;
#47940=DIRECTION ( 'NONE',  ( -0.1240347345892086200, 1.145860353393066553E-16, -0.9922778767136676281 ) ) ;
#47947=ORIENTED_EDGE ( 'NONE', *, *, #13142, .F. ) ;
#47973=EDGE_CURVE ( 'NONE', #38441, #22495, #8596, .T. ) ;
#48002=ORIENTED_EDGE ( 'NONE', *, *, #39529, .F. ) ;
#48034=DIRECTION ( 'NONE',  ( 1.000000000000000000, 2.866981220435666553E-17, 0.000000000000000000 ) ) ;
#48078=EDGE_CURVE ( 'NONE', #7144, #40267, #23864, .T. ) ;
#48084=VERTEX_POINT ( 'NONE', #31480 ) ;
#48105=LINE ( 'NONE', #14336, #20697 ) ;
#48111=PLANE ( 'NONE',  #8552 ) ;
#48121=CARTESIAN_POINT ( 'NONE',  ( -24.72409385541305582, -14.80920654474422271, 68.96470588235293064 ) ) ;
#48173=CARTESIAN_POINT ( 'NONE',  ( -50.42409385541305511, -14.80920654474410547, 56.99999999999998579 ) ) ;
#48175=CARTESIAN_POINT ( 'NONE',  ( -24.72409385541305582, -14.90920654474428630, 74.09999999999998010 ) ) ;
#48179=CARTESIAN_POINT ( 'NONE',  ( -24.72409385541305582, -15.80920654474410725, 65.99999999999998579 ) ) ;
#48180=ORIENTED_EDGE ( 'NONE', *, *, #31239, .T. ) ;
#48223=ORIENTED_EDGE ( 'NONE', *, *, #4136, .F. ) ;
#48224=CARTESIAN_POINT ( 'NONE',  ( -50.42609385541305755, -14.80920654474419074, 65.04705882352939739 ) ) ;
#48232=VERTEX_POINT ( 'NONE', #26516 ) ;
#48245=EDGE_CURVE ( 'NONE', #22914, #26590, #659, .T. ) ;
#48264=VECTOR ( 'NONE', #14580, 1000.000000000000000 ) ;
#48266=DIRECTION ( 'NONE',  ( 1.000000000000000000, 2.866981220435666553E-17, 0.000000000000000000 ) ) ;
#48340=AXIS2_PLACEMENT_3D ( 'NONE', #20207, #31781, #28077 ) ;
#48349=EDGE_CURVE ( 'NONE', #4839, #28413, #9929, .T. ) ;
#48363=ORIENTED_EDGE ( 'NONE', *, *, #25759, .F. ) ;
#48388=DIRECTION ( 'NONE',  ( -3.413470714839332458E-33, 1.190614954331866791E-16, -1.000000000000000000 ) ) ;
#48399=DIRECTION ( 'NONE',  ( -2.866981220435666553E-17, 1.000000000000000000, 1.190614954331866791E-16 ) ) ;
#48452=EDGE_CURVE ( 'NONE', #25220, #45934, #11140, .T. ) ;
#48486=PLANE ( 'NONE',  #31256 ) ;
#48502=VECTOR ( 'NONE', #40855, 1000.000000000000000 ) ;
#48552=EDGE_CURVE ( 'NONE', #1420, #10544, #19747, .T. ) ;
#48557=AXIS2_PLACEMENT_3D ( 'NONE', #19524, #31334, #46364 ) ;
#48562=DIRECTION ( 'NONE',  ( 1.000000000000000000, 2.866981220435666553E-17, 0.000000000000000000 ) ) ;
#48601=DIRECTION ( 'NONE',  ( 2.866981220435666553E-17, -1.000000000000000000, -1.190614954331866791E-16 ) ) ;
#48664=CARTESIAN_POINT ( 'NONE',  ( -41.79100562011894482, -14.90920654474422058, 68.06470588235292496 ) ) ;
#48695=EDGE_CURVE ( 'NONE', #48084, #42696, #10823, .T. ) ;
#48719=LINE ( 'NONE', #45065, #44674 ) ;
#48721=CARTESIAN_POINT ( 'NONE',  ( -50.42609385541305755, -14.90920654474415841, 62.92941176470587550 ) ) ;
ENDSEC;
END-ISO-10303-21;
